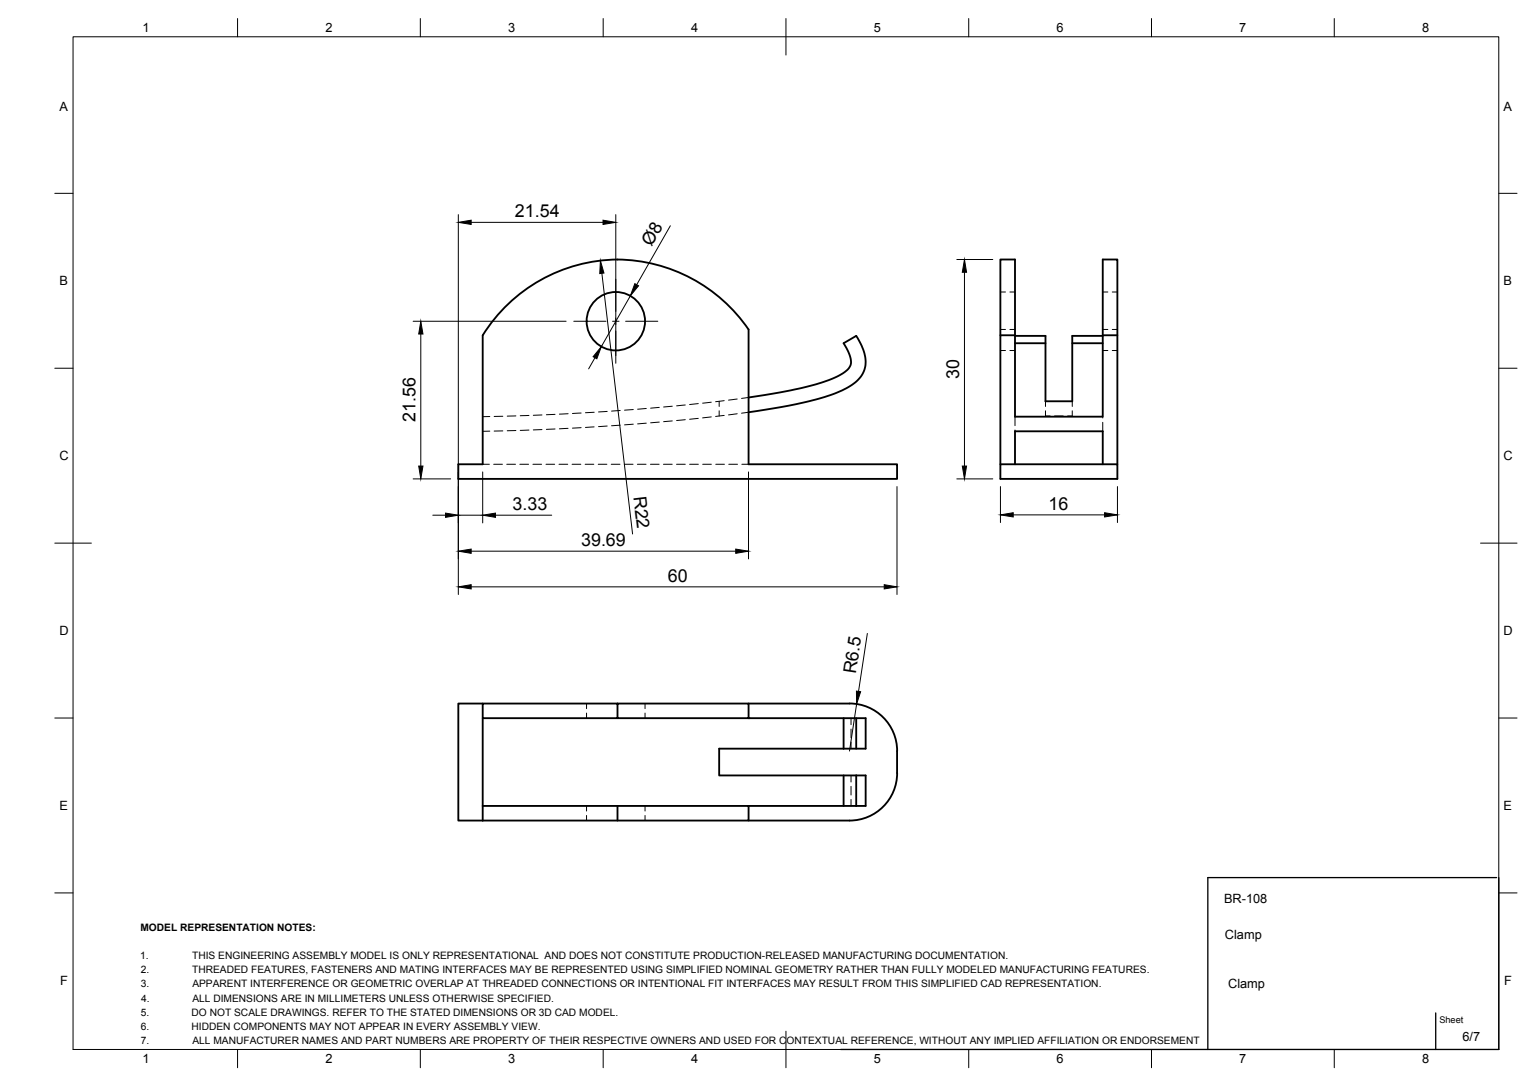
ISO-10303-21;
HEADER;
/* Generated by software containing ST-Developer
 * from STEP Tools, Inc. (www.steptools.com) 
 */

FILE_DESCRIPTION(
/* description */ (''),
/* implementation_level */ '2;1');

FILE_NAME(
/* name */ 'Clamp.step',
/* time_stamp */ '2026-11-14T03:52:36-08:00',
/* author */ (''),
/* organization */ (''),
/* preprocessor_version */ 'ST-DEVELOPER v20.2',
/* originating_system */ 'Autodesk Translation Framework v15.17.0.0',
/* authorisation */ '');

FILE_SCHEMA (('AUTOMOTIVE_DESIGN { 1 0 10303 214 3 1 1 }'));
ENDSEC;

DATA;
#10=MECHANICAL_DESIGN_GEOMETRIC_PRESENTATION_REPRESENTATION('',(#194),#19443);
#45=B_SPLINE_SURFACE_WITH_KNOTS('',5,1,((#10544,#10545),(#10546,#10547),
(#10548,#10549),(#10550,#10551),(#10552,#10553),(#10554,#10555),(#10556,
#10557),(#10558,#10559),(#10560,#10561),(#10562,#10563),(#10564,#10565),
(#10566,#10567),(#10568,#10569),(#10570,#10571),(#10572,#10573),(#10574,
#10575),(#10576,#10577),(#10578,#10579),(#10580,#10581),(#10582,#10583),
(#10584,#10585),(#10586,#10587),(#10588,#10589),(#10590,#10591),(#10592,
#10593)),.UNSPECIFIED.,.F.,.F.,.F.,(6,1,1,1,1,1,1,1,1,1,1,1,1,1,1,1,1,1,
1,1,6),(2,2),(0.,0.05,0.1,0.15,0.2,0.25,0.3,0.35,0.4,0.45,0.5,0.55,0.6,
0.65,0.7,0.75,0.8,0.85,0.9,0.95,0.997783576468117),(0.,2.28),
 .UNSPECIFIED.);
#46=B_SPLINE_SURFACE_WITH_KNOTS('',3,1,((#10795,#10796),(#10797,#10798),
(#10799,#10800),(#10801,#10802),(#10803,#10804),(#10805,#10806),(#10807,
#10808),(#10809,#10810),(#10811,#10812),(#10813,#10814),(#10815,#10816),
(#10817,#10818),(#10819,#10820),(#10821,#10822),(#10823,#10824),(#10825,
#10826),(#10827,#10828),(#10829,#10830),(#10831,#10832),(#10833,#10834),
(#10835,#10836),(#10837,#10838)),.UNSPECIFIED.,.F.,.F.,.F.,(4,3,3,3,3,3,
3,4),(2,2),(-1.,-0.911417181577933,-0.82714074028049,-0.742907558806874,
-0.633245293286216,-0.436057375062027,-0.250000004296482,-0.000486150394329065),
(0.,2.28),.UNSPECIFIED.);
#100=B_SPLINE_CURVE_WITH_KNOTS('',3,(#9842,#9843,#9844,#9845,#9846,#9847,
#9848,#9849,#9850,#9851,#9852,#9853,#9854,#9855,#9856,#9857,#9858,#9859,
#9860,#9861,#9862,#9863,#9864,#9865,#9866,#9867,#9868,#9869,#9870,#9871,
#9872,#9873,#9874,#9875,#9876,#9877,#9878,#9879,#9880,#9881,#9882,#9883,
#9884,#9885,#9886,#9887,#9888,#9889,#9890,#9891,#9892,#9893,#9894,#9895,
#9896,#9897,#9898,#9899,#9900,#9901,#9902,#9903,#9904,#9905,#9906,#9907,
#9908,#9909,#9910,#9911,#9912,#9913,#9914,#9915,#9916,#9917,#9918,#9919,
#9920,#9921,#9922,#9923),.UNSPECIFIED.,.F.,.F.,(4,3,3,3,3,3,3,3,3,3,3,3,
3,3,3,3,3,3,3,3,3,3,3,3,3,3,3,4),(-2.06741991825068,-1.98285131338516,-1.88559013949774,
-1.77615559465644,-1.68790443753717,-1.60974818243148,-1.53676333066918,
-1.46730179083953,-1.4010195987632,-1.3378649598913,-1.27712721666041,-1.21746070099515,
-1.15761317028239,-1.09756920913897,-1.03668973178852,-0.971602936806244,
-0.902947147892858,-0.830652039518071,-0.754808243576467,-0.676131879378777,
-0.596648141755566,-0.518810466257096,-0.437949267560199,-0.352276201339158,
-0.261252153029477,-0.169810646360919,-0.0802964651905899,0.),
 .UNSPECIFIED.);
#101=B_SPLINE_CURVE_WITH_KNOTS('',3,(#9927,#9928,#9929,#9930,#9931,#9932,
#9933,#9934,#9935,#9936,#9937,#9938,#9939,#9940,#9941,#9942,#9943,#9944,
#9945,#9946,#9947,#9948,#9949,#9950,#9951,#9952,#9953,#9954,#9955,#9956,
#9957,#9958,#9959,#9960,#9961,#9962,#9963,#9964,#9965,#9966,#9967,#9968,
#9969,#9970,#9971,#9972,#9973,#9974,#9975,#9976,#9977,#9978,#9979,#9980,
#9981,#9982,#9983,#9984,#9985,#9986,#9987,#9988,#9989,#9990,#9991,#9992,
#9993,#9994,#9995,#9996,#9997,#9998,#9999,#10000,#10001,#10002,#10003,#10004,
#10005,#10006,#10007,#10008,#10009,#10010,#10011,#10012,#10013,#10014,#10015,
#10016,#10017,#10018,#10019,#10020,#10021,#10022,#10023,#10024,#10025,#10026,
#10027,#10028,#10029,#10030,#10031,#10032,#10033,#10034,#10035,#10036,#10037,
#10038,#10039,#10040,#10041,#10042,#10043,#10044,#10045,#10046,#10047,#10048,
#10049,#10050,#10051,#10052,#10053,#10054,#10055,#10056,#10057,#10058,#10059,
#10060,#10061,#10062,#10063,#10064,#10065,#10066,#10067,#10068,#10069,#10070,
#10071,#10072,#10073,#10074,#10075,#10076,#10077,#10078,#10079,#10080,#10081,
#10082,#10083,#10084,#10085,#10086,#10087,#10088,#10089,#10090,#10091,#10092,
#10093,#10094,#10095,#10096,#10097,#10098,#10099,#10100,#10101,#10102,#10103,
#10104,#10105,#10106,#10107,#10108,#10109,#10110,#10111,#10112,#10113,#10114,
#10115,#10116,#10117,#10118,#10119,#10120,#10121,#10122,#10123,#10124,#10125,
#10126,#10127,#10128,#10129,#10130,#10131,#10132,#10133,#10134,#10135,#10136,
#10137,#10138,#10139,#10140,#10141,#10142,#10143,#10144,#10145,#10146,#10147,
#10148,#10149),.UNSPECIFIED.,.F.,.F.,(4,3,3,3,3,3,3,3,3,3,3,3,3,3,3,3,3,
3,3,3,3,3,3,3,3,3,3,3,3,3,3,3,3,3,3,3,3,3,3,3,3,3,3,3,3,3,3,3,3,3,3,3,3,
3,3,3,3,3,3,3,3,3,3,3,3,3,3,3,3,3,3,3,3,3,4),(-5.48556059930356,-5.3742901434944,
-5.26503542580367,-5.1577836872572,-5.04847386928929,-4.94641423339456,
-4.84632584686655,-4.74823870879311,-4.65217176427579,-4.55995510908532,
-4.49079261769247,-4.48335167319748,-4.47546446159234,-4.42482571833493,
-4.37539535138974,-4.32789456523567,-4.28330514351393,-4.22386198589148,
-4.16367959879141,-4.11102001007885,-4.0879814400171,-4.07451117436979,
-4.06881777499082,-4.06396069374141,-4.01960604117804,-3.97171900412971,
-3.91910957291902,-3.86588690476172,-3.81609285440557,-3.7976703630769,
-3.7838534945804,-3.78018597444469,-3.74240288909089,-3.68720132020267,
-3.63214582482016,-3.58397226636046,-3.54161995271181,-3.50476212826565,
-3.48863683007046,-3.48328860908609,-3.47990706616965,-3.42477351581283,
-3.36626643116087,-3.30651189415172,-3.25207197124738,-3.24675735714258,
-3.20212792397615,-3.15620343761748,-3.10888467447819,-3.06005777462237,
-3.00959125336058,-2.9774459670657,-2.96187559401661,-2.95363335797171,
-2.94977181559791,-2.80448949951976,-2.65815449920403,-2.51096234105158,
-2.36291829657365,-2.21466098559846,-2.06653880208347,-1.98094209192433,
-1.80620872497199,-1.61914703673255,-1.40683918645954,-1.18478189892939,
-1.00215186108193,-0.839832576136721,-0.690457992737357,-0.550511129775,
-0.421119097329167,-0.296518986825456,-0.178327808264077,-0.0898716726840916,
-0.0508038206324297),.UNSPECIFIED.);
#102=B_SPLINE_CURVE_WITH_KNOTS('',3,(#10159,#10160,#10161,#10162,#10163,
#10164,#10165,#10166,#10167,#10168,#10169,#10170,#10171,#10172,#10173,#10174,
#10175,#10176,#10177,#10178,#10179,#10180,#10181,#10182,#10183,#10184,#10185,
#10186,#10187,#10188,#10189,#10190,#10191,#10192,#10193,#10194,#10195,#10196,
#10197,#10198,#10199,#10200,#10201,#10202,#10203,#10204,#10205,#10206,#10207,
#10208,#10209,#10210,#10211,#10212,#10213,#10214,#10215,#10216,#10217,#10218,
#10219,#10220,#10221,#10222,#10223,#10224,#10225,#10226,#10227,#10228,#10229,
#10230,#10231,#10232,#10233,#10234,#10235,#10236,#10237,#10238,#10239,#10240,
#10241,#10242,#10243,#10244,#10245,#10246,#10247,#10248,#10249,#10250,#10251,
#10252,#10253,#10254,#10255,#10256,#10257,#10258,#10259,#10260,#10261,#10262,
#10263,#10264,#10265,#10266,#10267,#10268,#10269,#10270,#10271,#10272,#10273,
#10274,#10275,#10276,#10277,#10278,#10279,#10280,#10281,#10282,#10283,#10284,
#10285,#10286,#10287,#10288,#10289,#10290,#10291,#10292,#10293,#10294,#10295,
#10296,#10297,#10298,#10299,#10300,#10301,#10302,#10303,#10304,#10305,#10306),
 .UNSPECIFIED.,.F.,.F.,(4,3,3,3,3,3,3,3,3,3,3,3,3,3,3,3,3,3,3,3,3,3,3,3,
3,3,3,3,3,3,3,3,3,3,3,3,3,3,3,3,3,3,3,3,3,3,3,3,3,4),(-9.10855960492281,
-8.53921958763157,-8.00869400174604,-7.76001013336219,-7.63955388461377,
-7.56405433243604,-7.52369479269779,-7.50080752596703,-7.07650861767828,
-6.72947065932967,-6.625116589863,-6.56600757594707,-6.53309864263095,-6.50820482569483,
-6.14678803531956,-5.8044120104252,-5.71451198234767,-5.68978334933782,
-5.67339715853821,-5.3117835102232,-4.98297267917569,-4.82884260212217,
-4.75418584604937,-4.72996428359645,-4.70456344497697,-4.32299778199833,
-3.91934735473528,-3.47804282231225,-3.37094180328571,-3.35701328282335,
-3.17572752382557,-2.99394470365639,-2.80883622817471,-2.61893869722417,
-2.42004735513258,-2.20439292822488,-1.94398198484001,-1.70733551341788,
-1.50026985092353,-1.31908739624096,-1.16055274839372,-1.01261022609456,
-0.870637451570371,-0.733373124428186,-0.599882166408188,-0.4695171211688,
-0.342516273201481,-0.216889573446191,-0.0922346720977524,-0.0508102134630154),
 .UNSPECIFIED.);
#103=B_SPLINE_CURVE_WITH_KNOTS('',3,(#10309,#10310,#10311,#10312,#10313,
#10314,#10315,#10316,#10317,#10318,#10319,#10320,#10321,#10322,#10323,#10324,
#10325,#10326,#10327,#10328,#10329,#10330,#10331,#10332,#10333,#10334,#10335,
#10336,#10337,#10338,#10339,#10340,#10341,#10342,#10343,#10344,#10345,#10346,
#10347,#10348,#10349,#10350,#10351,#10352,#10353,#10354,#10355,#10356,#10357,
#10358,#10359,#10360,#10361,#10362,#10363,#10364,#10365,#10366,#10367,#10368,
#10369,#10370,#10371,#10372,#10373,#10374,#10375,#10376,#10377,#10378,#10379,
#10380,#10381,#10382,#10383,#10384,#10385,#10386,#10387,#10388,#10389,#10390,
#10391,#10392,#10393,#10394,#10395,#10396,#10397,#10398,#10399,#10400,#10401,
#10402,#10403,#10404,#10405,#10406,#10407,#10408,#10409,#10410,#10411,#10412,
#10413,#10414,#10415,#10416,#10417,#10418,#10419,#10420,#10421,#10422,#10423,
#10424,#10425,#10426,#10427,#10428,#10429,#10430,#10431,#10432,#10433,#10434,
#10435,#10436,#10437,#10438,#10439,#10440,#10441,#10442,#10443,#10444,#10445,
#10446,#10447,#10448,#10449,#10450,#10451,#10452,#10453,#10454,#10455,#10456,
#10457,#10458,#10459,#10460,#10461,#10462,#10463,#10464,#10465,#10466,#10467,
#10468,#10469,#10470,#10471,#10472,#10473,#10474,#10475,#10476,#10477,#10478,
#10479,#10480,#10481,#10482,#10483,#10484,#10485,#10486,#10487,#10488,#10489,
#10490,#10491,#10492,#10493,#10494,#10495,#10496,#10497,#10498,#10499,#10500,
#10501,#10502,#10503,#10504,#10505,#10506,#10507,#10508,#10509,#10510,#10511,
#10512,#10513,#10514,#10515,#10516,#10517,#10518,#10519,#10520,#10521,#10522,
#10523,#10524,#10525,#10526,#10527,#10528,#10529,#10530,#10531,#10532,#10533,
#10534,#10535,#10536,#10537,#10538,#10539,#10540,#10541,#10542,#10543),
 .UNSPECIFIED.,.F.,.F.,(4,3,3,3,3,3,3,3,3,3,3,3,3,3,3,3,3,3,3,3,3,3,3,3,
3,3,3,3,3,3,3,3,3,3,3,3,3,3,3,3,3,3,3,3,3,3,3,3,3,3,3,3,3,3,3,3,3,3,3,3,
3,3,3,3,3,3,3,3,3,3,3,3,3,3,3,3,3,3,4),(-2.02127869660357,-1.98943301980102,
-1.90463341590351,-1.81753768881889,-1.72704367650355,-1.63130693910596,
-1.51951582960439,-1.38310822332673,-1.26646899428466,-1.24459913883927,
-1.23346627262239,-1.22758843562283,-1.22207812234324,-1.15025709426344,
-1.08179540629444,-1.01496797201,-0.950320490610193,-0.916551307158433,
-0.853832223783638,-0.792204136679497,-0.731660192212863,-0.672186959028124,
-0.613766411128121,-0.590013602117237,-0.579621748174975,-0.57475056663954,
-0.571134341312111,-0.569460165760368,-0.547675695632619,-0.526546111795004,
-0.506025620571326,-0.485455200188757,-0.466281411555601,-0.447521496264729,
-0.429320222384578,-0.42374393904105,-0.399392451378572,-0.374499279646305,
-0.361614191206241,-0.358455047560918,-0.356511913591946,-0.35473329500815,
-0.344318954647855,-0.334029402325209,-0.323701337929739,-0.313256768851862,
-0.302559895706747,-0.291964358202782,-0.281691465164288,-0.279957855794893,
-0.278600543326745,-0.271418572125793,-0.262582752193856,-0.253672103340293,
-0.245540273158529,-0.238031151837375,-0.230909539922171,-0.226625838952106,
-0.216671112747294,-0.205500677732474,-0.193363451631138,-0.179480016034121,
-0.176626080324589,-0.166163697812807,-0.160971082256157,-0.159162329434394,
-0.157259342194023,-0.144809310782755,-0.13207070022678,-0.119040767714878,
-0.10571865453773,-0.091955933688298,-0.0779231319105442,-0.0636219003870916,
-0.0490527186804175,-0.034085309706883,-0.0188794529916116,-0.00332468735320998,
0.),.UNSPECIFIED.);
#104=B_SPLINE_CURVE_WITH_KNOTS('',5,(#10597,#10598,#10599,#10600,#10601,
#10602,#10603,#10604,#10605,#10606,#10607,#10608,#10609,#10610,#10611,#10612),
 .UNSPECIFIED.,.F.,.F.,(6,1,1,1,1,1,1,1,1,1,1,6),(0.481836522428161,0.5,
0.55,0.6,0.65,0.7,0.75,0.8,0.85,0.9,0.95,0.997783576468117),
 .UNSPECIFIED.);
#105=B_SPLINE_CURVE_WITH_KNOTS('',5,(#10614,#10615,#10616,#10617,#10618,
#10619,#10620,#10621,#10622,#10623,#10624,#10625,#10626,#10627,#10628),
 .UNSPECIFIED.,.F.,.F.,(6,1,1,1,1,1,1,1,1,1,6),(0.,0.05,0.1,0.15,0.2,0.25,
0.3,0.35,0.4,0.45,0.481836522428277),.UNSPECIFIED.);
#106=B_SPLINE_CURVE_WITH_KNOTS('',3,(#10632,#10633,#10634,#10635,#10636,
#10637,#10638,#10639,#10640,#10641,#10642,#10643,#10644,#10645,#10646,#10647,
#10648,#10649,#10650,#10651,#10652,#10653,#10654,#10655,#10656,#10657,#10658,
#10659,#10660,#10661,#10662,#10663,#10664,#10665,#10666,#10667,#10668,#10669,
#10670,#10671,#10672,#10673,#10674,#10675,#10676,#10677,#10678,#10679,#10680,
#10681,#10682,#10683,#10684,#10685,#10686,#10687,#10688,#10689,#10690,#10691,
#10692,#10693,#10694,#10695),.UNSPECIFIED.,.F.,.F.,(4,3,3,3,3,3,3,3,3,3,
3,3,3,3,3,3,3,3,3,3,3,4),(-0.481836522428277,-0.45532349494856,-0.432546979219204,
-0.411758376367504,-0.392204877029118,-0.373446283655192,-0.35531022111101,
-0.337405801369786,-0.319166348359288,-0.3005346337047,-0.281334526323306,
-0.261758757819788,-0.241752343726884,-0.221237113369723,-0.200124506192356,
-0.178341717407575,-0.155289187104983,-0.131213486522262,-0.105793029252951,
-0.0769868283461338,-0.0445183707397895,0.),.UNSPECIFIED.);
#107=B_SPLINE_CURVE_WITH_KNOTS('',3,(#10697,#10698,#10699,#10700,#10701,
#10702,#10703,#10704,#10705,#10706,#10707,#10708,#10709,#10710,#10711,#10712,
#10713,#10714,#10715,#10716,#10717,#10718,#10719,#10720,#10721,#10722,#10723,
#10724,#10725,#10726,#10727,#10728,#10729,#10730,#10731,#10732,#10733,#10734,
#10735,#10736,#10737,#10738,#10739,#10740,#10741,#10742,#10743,#10744,#10745,
#10746,#10747,#10748,#10749,#10750,#10751,#10752,#10753,#10754,#10755,#10756,
#10757,#10758,#10759,#10760,#10761,#10762,#10763,#10764,#10765,#10766,#10767,
#10768,#10769,#10770,#10771,#10772),.UNSPECIFIED.,.F.,.F.,(4,3,3,3,3,3,
3,3,3,3,3,3,3,3,3,3,3,3,3,3,3,3,3,3,3,4),(-1.78233413254146,-1.68011036101728,
-1.59770235095047,-1.52404961693638,-1.45502228044773,-1.38923460267853,
-1.3265205751834,-1.26669886884287,-1.20909993484359,-1.15227786115506,
-1.09526869988759,-1.03807287674761,-0.979856117355335,-0.917508293433697,
-0.851705632256396,-0.782466326919254,-0.709863093111388,-0.634726037442554,
-0.555385282762235,-0.481050928781323,-0.403338688398482,-0.320930918924746,
-0.234066753872441,-0.147080803661418,-0.0621010514640444,0.),
 .UNSPECIFIED.);
#108=B_SPLINE_CURVE_WITH_KNOTS('',3,(#10782,#10783,#10784,#10785,#10786,
#10787,#10788,#10789,#10790,#10791,#10792,#10793),.UNSPECIFIED.,.F.,.F.,
(4,2,2,2,2,4),(-8.5482923307436,-7.74150904834439,-6.97394683763538,-6.20677862322595,
-5.20801064419706,-3.86462956150548),.UNSPECIFIED.);
#109=B_SPLINE_CURVE_WITH_KNOTS('',3,(#10841,#10842,#10843,#10844,#10845,
#10846,#10847,#10848),.UNSPECIFIED.,.F.,.F.,(4,2,2,4),(0.000486150394328964,
0.250000004296481,0.436057375062024,0.485741739397154),.UNSPECIFIED.);
#110=B_SPLINE_CURVE_WITH_KNOTS('',3,(#10852,#10853,#10854,#10855,#10856,
#10857,#10858,#10859),.UNSPECIFIED.,.F.,.F.,(4,2,2,4),(-0.485741739388686,
-0.436057375062167,-0.250000004296568,-0.000486150394336471),
 .UNSPECIFIED.);
#111=B_SPLINE_CURVE_WITH_KNOTS('',3,(#10860,#10861,#10862,#10863,#10864,
#10865,#10866,#10867,#10868,#10869,#10870,#10871),.UNSPECIFIED.,.F.,.F.,
(4,2,2,2,2,4),(-1.,-0.911417181577934,-0.82714074028049,-0.742907558806875,
-0.633245293286218,-0.485745357261071),.UNSPECIFIED.);
#178=SHAPE_REPRESENTATION_RELATIONSHIP('SRR','None',#19478,#186);
#186=ADVANCED_BREP_SHAPE_REPRESENTATION('',(#202),#19438);
#194=STYLED_ITEM('',(#19525),#202);
#202=MANIFOLD_SOLID_BREP('Body1',#2021);
#210=FACE_BOUND('',#410,.T.);
#211=FACE_BOUND('',#414,.T.);
#212=FACE_BOUND('',#420,.T.);
#213=FACE_BOUND('',#427,.T.);
#227=PLANE('',#2154);
#228=PLANE('',#2158);
#229=PLANE('',#2159);
#230=PLANE('',#2160);
#231=PLANE('',#2161);
#232=PLANE('',#2162);
#233=PLANE('',#2163);
#234=PLANE('',#2164);
#235=PLANE('',#2165);
#236=PLANE('',#2166);
#237=PLANE('',#2167);
#238=PLANE('',#2168);
#239=PLANE('',#2172);
#240=PLANE('',#2173);
#241=PLANE('',#2174);
#242=PLANE('',#2181);
#243=PLANE('',#2182);
#244=PLANE('',#2186);
#245=PLANE('',#2187);
#246=PLANE('',#2194);
#295=FACE_OUTER_BOUND('',#394,.T.);
#296=FACE_OUTER_BOUND('',#395,.T.);
#297=FACE_OUTER_BOUND('',#396,.T.);
#298=FACE_OUTER_BOUND('',#397,.T.);
#299=FACE_OUTER_BOUND('',#398,.T.);
#300=FACE_OUTER_BOUND('',#399,.T.);
#301=FACE_OUTER_BOUND('',#400,.T.);
#302=FACE_OUTER_BOUND('',#401,.T.);
#303=FACE_OUTER_BOUND('',#402,.T.);
#304=FACE_OUTER_BOUND('',#403,.T.);
#305=FACE_OUTER_BOUND('',#404,.T.);
#306=FACE_OUTER_BOUND('',#405,.T.);
#307=FACE_OUTER_BOUND('',#406,.T.);
#308=FACE_OUTER_BOUND('',#407,.T.);
#309=FACE_OUTER_BOUND('',#408,.T.);
#310=FACE_OUTER_BOUND('',#409,.T.);
#311=FACE_OUTER_BOUND('',#411,.T.);
#312=FACE_OUTER_BOUND('',#412,.T.);
#313=FACE_OUTER_BOUND('',#413,.T.);
#314=FACE_OUTER_BOUND('',#415,.T.);
#315=FACE_OUTER_BOUND('',#416,.T.);
#316=FACE_OUTER_BOUND('',#417,.T.);
#317=FACE_OUTER_BOUND('',#418,.T.);
#318=FACE_OUTER_BOUND('',#419,.T.);
#319=FACE_OUTER_BOUND('',#421,.T.);
#320=FACE_OUTER_BOUND('',#422,.T.);
#321=FACE_OUTER_BOUND('',#423,.T.);
#322=FACE_OUTER_BOUND('',#424,.T.);
#323=FACE_OUTER_BOUND('',#425,.T.);
#324=FACE_OUTER_BOUND('',#426,.T.);
#394=EDGE_LOOP('',(#1437,#1438,#1439,#1440));
#395=EDGE_LOOP('',(#1441,#1442,#1443,#1444,#1445,#1446));
#396=EDGE_LOOP('',(#1447,#1448,#1449,#1450));
#397=EDGE_LOOP('',(#1451,#1452,#1453,#1454));
#398=EDGE_LOOP('',(#1455,#1456,#1457,#1458,#1459,#1460,#1461,#1462,#1463,
#1464,#1465,#1466,#1467,#1468));
#399=EDGE_LOOP('',(#1469,#1470,#1471,#1472));
#400=EDGE_LOOP('',(#1473,#1474,#1475,#1476));
#401=EDGE_LOOP('',(#1477,#1478,#1479,#1480));
#402=EDGE_LOOP('',(#1481,#1482,#1483,#1484));
#403=EDGE_LOOP('',(#1485,#1486,#1487,#1488,#1489,#1490,#1491,#1492,#1493,
#1494));
#404=EDGE_LOOP('',(#1495,#1496,#1497,#1498));
#405=EDGE_LOOP('',(#1499,#1500,#1501,#1502));
#406=EDGE_LOOP('',(#1503,#1504,#1505,#1506,#1507,#1508,#1509,#1510,#1511,
#1512));
#407=EDGE_LOOP('',(#1513,#1514,#1515,#1516));
#408=EDGE_LOOP('',(#1517,#1518,#1519,#1520));
#409=EDGE_LOOP('',(#1521,#1522,#1523,#1524,#1525));
#410=EDGE_LOOP('',(#1526));
#411=EDGE_LOOP('',(#1527,#1528,#1529,#1530));
#412=EDGE_LOOP('',(#1531,#1532,#1533,#1534,#1535,#1536));
#413=EDGE_LOOP('',(#1537,#1538,#1539,#1540,#1541,#1542,#1543,#1544,#1545));
#414=EDGE_LOOP('',(#1546));
#415=EDGE_LOOP('',(#1547,#1548,#1549,#1550));
#416=EDGE_LOOP('',(#1551,#1552,#1553,#1554));
#417=EDGE_LOOP('',(#1555,#1556,#1557,#1558));
#418=EDGE_LOOP('',(#1559,#1560,#1561,#1562));
#419=EDGE_LOOP('',(#1563,#1564,#1565,#1566,#1567));
#420=EDGE_LOOP('',(#1568));
#421=EDGE_LOOP('',(#1569,#1570,#1571,#1572,#1573,#1574,#1575,#1576,#1577,
#1578,#1579,#1580));
#422=EDGE_LOOP('',(#1581,#1582,#1583,#1584,#1585,#1586));
#423=EDGE_LOOP('',(#1587,#1588,#1589,#1590));
#424=EDGE_LOOP('',(#1591,#1592,#1593,#1594));
#425=EDGE_LOOP('',(#1595,#1596,#1597,#1598));
#426=EDGE_LOOP('',(#1599,#1600,#1601,#1602,#1603,#1604,#1605,#1606,#1607));
#427=EDGE_LOOP('',(#1608));
#489=LINE('',#9792,#616);
#490=LINE('',#9795,#617);
#491=LINE('',#9798,#618);
#492=LINE('',#9802,#619);
#493=LINE('',#9804,#620);
#494=LINE('',#9805,#621);
#495=LINE('',#9808,#622);
#496=LINE('',#9811,#623);
#497=LINE('',#9813,#624);
#498=LINE('',#9817,#625);
#499=LINE('',#9818,#626);
#500=LINE('',#9820,#627);
#501=LINE('',#9822,#628);
#502=LINE('',#9824,#629);
#503=LINE('',#9826,#630);
#504=LINE('',#9828,#631);
#505=LINE('',#9830,#632);
#506=LINE('',#9832,#633);
#507=LINE('',#9834,#634);
#508=LINE('',#9835,#635);
#509=LINE('',#9837,#636);
#510=LINE('',#9838,#637);
#511=LINE('',#9925,#638);
#512=LINE('',#10150,#639);
#513=LINE('',#10153,#640);
#514=LINE('',#10155,#641);
#515=LINE('',#10156,#642);
#516=LINE('',#10308,#643);
#517=LINE('',#10595,#644);
#518=LINE('',#10630,#645);
#519=LINE('',#10773,#646);
#520=LINE('',#10776,#647);
#521=LINE('',#10777,#648);
#522=LINE('',#10780,#649);
#523=LINE('',#10794,#650);
#524=LINE('',#10839,#651);
#525=LINE('',#10850,#652);
#526=LINE('',#10874,#653);
#527=LINE('',#10877,#654);
#528=LINE('',#10882,#655);
#529=LINE('',#10886,#656);
#530=LINE('',#10887,#657);
#531=LINE('',#10890,#658);
#532=LINE('',#10891,#659);
#533=LINE('',#10894,#660);
#534=LINE('',#10901,#661);
#535=LINE('',#10903,#662);
#536=LINE('',#10905,#663);
#537=LINE('',#10907,#664);
#538=LINE('',#10908,#665);
#539=LINE('',#10911,#666);
#540=LINE('',#10916,#667);
#541=LINE('',#10921,#668);
#542=LINE('',#10922,#669);
#543=LINE('',#10925,#670);
#544=LINE('',#10926,#671);
#545=LINE('',#10930,#672);
#546=LINE('',#10934,#673);
#616=VECTOR('',#2353,10.);
#617=VECTOR('',#2356,10.);
#618=VECTOR('',#2359,10.);
#619=VECTOR('',#2362,10.);
#620=VECTOR('',#2363,10.);
#621=VECTOR('',#2364,10.);
#622=VECTOR('',#2367,10.);
#623=VECTOR('',#2370,10.);
#624=VECTOR('',#2373,10.);
#625=VECTOR('',#2376,10.);
#626=VECTOR('',#2377,10.);
#627=VECTOR('',#2378,10.);
#628=VECTOR('',#2379,10.);
#629=VECTOR('',#2380,10.);
#630=VECTOR('',#2381,10.);
#631=VECTOR('',#2382,10.);
#632=VECTOR('',#2383,10.);
#633=VECTOR('',#2384,10.);
#634=VECTOR('',#2385,10.);
#635=VECTOR('',#2386,10.);
#636=VECTOR('',#2389,10.);
#637=VECTOR('',#2390,10.);
#638=VECTOR('',#2393,10.);
#639=VECTOR('',#2394,10.);
#640=VECTOR('',#2397,10.);
#641=VECTOR('',#2398,10.);
#642=VECTOR('',#2399,10.);
#643=VECTOR('',#2402,10.);
#644=VECTOR('',#2403,10.);
#645=VECTOR('',#2404,10.);
#646=VECTOR('',#2405,10.);
#647=VECTOR('',#2408,10.);
#648=VECTOR('',#2409,10.);
#649=VECTOR('',#2412,10.);
#650=VECTOR('',#2413,10.);
#651=VECTOR('',#2414,10.);
#652=VECTOR('',#2415,10.);
#653=VECTOR('',#2420,10.);
#654=VECTOR('',#2423,10.);
#655=VECTOR('',#2428,10.);
#656=VECTOR('',#2433,10.);
#657=VECTOR('',#2434,10.);
#658=VECTOR('',#2437,10.);
#659=VECTOR('',#2438,10.);
#660=VECTOR('',#2441,10.);
#661=VECTOR('',#2450,3.99999999999997);
#662=VECTOR('',#2453,10.);
#663=VECTOR('',#2456,10.);
#664=VECTOR('',#2459,10.);
#665=VECTOR('',#2460,10.);
#666=VECTOR('',#2463,10.);
#667=VECTOR('',#2468,10.);
#668=VECTOR('',#2473,10.);
#669=VECTOR('',#2474,10.);
#670=VECTOR('',#2477,10.);
#671=VECTOR('',#2478,10.);
#672=VECTOR('',#2483,3.99999999999997);
#673=VECTOR('',#2488,10.);
#743=CIRCLE('',#2152,6.5);
#744=CIRCLE('',#2153,6.5);
#745=CIRCLE('',#2155,6.5);
#746=CIRCLE('',#2157,6.5);
#747=CIRCLE('',#2169,22.);
#748=CIRCLE('',#2170,22.);
#749=CIRCLE('',#2171,3.99999999999997);
#750=CIRCLE('',#2175,22.);
#751=CIRCLE('',#2176,22.);
#752=CIRCLE('',#2177,3.99999999999997);
#753=CIRCLE('',#2183,22.);
#754=CIRCLE('',#2184,22.);
#755=CIRCLE('',#2185,3.99999999999997);
#756=CIRCLE('',#2189,3.99999999999997);
#757=CIRCLE('',#2191,22.);
#758=CIRCLE('',#2193,22.);
#834=VERTEX_POINT('',#9788);
#835=VERTEX_POINT('',#9789);
#836=VERTEX_POINT('',#9791);
#837=VERTEX_POINT('',#9793);
#838=VERTEX_POINT('',#9797);
#839=VERTEX_POINT('',#9799);
#840=VERTEX_POINT('',#9801);
#841=VERTEX_POINT('',#9803);
#842=VERTEX_POINT('',#9807);
#843=VERTEX_POINT('',#9809);
#844=VERTEX_POINT('',#9815);
#845=VERTEX_POINT('',#9816);
#846=VERTEX_POINT('',#9819);
#847=VERTEX_POINT('',#9821);
#848=VERTEX_POINT('',#9823);
#849=VERTEX_POINT('',#9825);
#850=VERTEX_POINT('',#9827);
#851=VERTEX_POINT('',#9829);
#852=VERTEX_POINT('',#9831);
#853=VERTEX_POINT('',#9833);
#854=VERTEX_POINT('',#9840);
#855=VERTEX_POINT('',#9841);
#856=VERTEX_POINT('',#9924);
#857=VERTEX_POINT('',#9926);
#858=VERTEX_POINT('',#10152);
#859=VERTEX_POINT('',#10154);
#860=VERTEX_POINT('',#10158);
#861=VERTEX_POINT('',#10307);
#862=VERTEX_POINT('',#10594);
#863=VERTEX_POINT('',#10596);
#864=VERTEX_POINT('',#10613);
#865=VERTEX_POINT('',#10629);
#866=VERTEX_POINT('',#10631);
#867=VERTEX_POINT('',#10696);
#868=VERTEX_POINT('',#10775);
#869=VERTEX_POINT('',#10779);
#870=VERTEX_POINT('',#10781);
#871=VERTEX_POINT('',#10840);
#872=VERTEX_POINT('',#10849);
#873=VERTEX_POINT('',#10851);
#874=VERTEX_POINT('',#10876);
#875=VERTEX_POINT('',#10878);
#876=VERTEX_POINT('',#10880);
#877=VERTEX_POINT('',#10883);
#878=VERTEX_POINT('',#10889);
#879=VERTEX_POINT('',#10893);
#880=VERTEX_POINT('',#10895);
#881=VERTEX_POINT('',#10898);
#882=VERTEX_POINT('',#10910);
#883=VERTEX_POINT('',#10912);
#884=VERTEX_POINT('',#10914);
#885=VERTEX_POINT('',#10917);
#886=VERTEX_POINT('',#10920);
#887=VERTEX_POINT('',#10924);
#888=VERTEX_POINT('',#10928);
#889=VERTEX_POINT('',#10932);
#1067=EDGE_CURVE('',#834,#835,#743,.T.);
#1068=EDGE_CURVE('',#835,#836,#489,.T.);
#1069=EDGE_CURVE('',#836,#837,#744,.T.);
#1070=EDGE_CURVE('',#837,#834,#490,.T.);
#1071=EDGE_CURVE('',#834,#838,#491,.T.);
#1072=EDGE_CURVE('',#839,#838,#745,.T.);
#1073=EDGE_CURVE('',#839,#840,#492,.T.);
#1074=EDGE_CURVE('',#841,#840,#493,.T.);
#1075=EDGE_CURVE('',#835,#841,#494,.T.);
#1076=EDGE_CURVE('',#838,#842,#495,.T.);
#1077=EDGE_CURVE('',#842,#843,#746,.T.);
#1078=EDGE_CURVE('',#843,#839,#496,.T.);
#1079=EDGE_CURVE('',#837,#842,#497,.T.);
#1080=EDGE_CURVE('',#844,#845,#498,.T.);
#1081=EDGE_CURVE('',#845,#843,#499,.T.);
#1082=EDGE_CURVE('',#846,#836,#500,.T.);
#1083=EDGE_CURVE('',#846,#847,#501,.T.);
#1084=EDGE_CURVE('',#848,#847,#502,.T.);
#1085=EDGE_CURVE('',#848,#849,#503,.T.);
#1086=EDGE_CURVE('',#850,#849,#504,.T.);
#1087=EDGE_CURVE('',#851,#850,#505,.T.);
#1088=EDGE_CURVE('',#851,#852,#506,.T.);
#1089=EDGE_CURVE('',#852,#853,#507,.T.);
#1090=EDGE_CURVE('',#844,#853,#508,.T.);
#1091=EDGE_CURVE('',#841,#850,#509,.T.);
#1092=EDGE_CURVE('',#840,#851,#510,.T.);
#1093=EDGE_CURVE('',#854,#855,#100,.T.);
#1094=EDGE_CURVE('',#854,#856,#511,.T.);
#1095=EDGE_CURVE('',#857,#856,#101,.T.);
#1096=EDGE_CURVE('',#855,#857,#512,.T.);
#1097=EDGE_CURVE('',#858,#854,#513,.T.);
#1098=EDGE_CURVE('',#858,#859,#514,.T.);
#1099=EDGE_CURVE('',#856,#859,#515,.T.);
#1100=EDGE_CURVE('',#860,#858,#102,.T.);
#1101=EDGE_CURVE('',#861,#860,#516,.T.);
#1102=EDGE_CURVE('',#859,#861,#103,.T.);
#1103=EDGE_CURVE('',#855,#862,#517,.T.);
#1104=EDGE_CURVE('',#863,#862,#104,.T.);
#1105=EDGE_CURVE('',#864,#863,#105,.T.);
#1106=EDGE_CURVE('',#865,#864,#518,.T.);
#1107=EDGE_CURVE('',#866,#865,#106,.T.);
#1108=EDGE_CURVE('',#866,#867,#107,.T.);
#1109=EDGE_CURVE('',#867,#860,#519,.T.);
#1110=EDGE_CURVE('',#857,#868,#520,.T.);
#1111=EDGE_CURVE('',#862,#868,#521,.T.);
#1112=EDGE_CURVE('',#866,#869,#522,.T.);
#1113=EDGE_CURVE('',#870,#869,#108,.T.);
#1114=EDGE_CURVE('',#867,#870,#523,.T.);
#1115=EDGE_CURVE('',#870,#861,#524,.T.);
#1116=EDGE_CURVE('',#871,#869,#109,.T.);
#1117=EDGE_CURVE('',#871,#872,#525,.T.);
#1118=EDGE_CURVE('',#873,#872,#110,.T.);
#1119=EDGE_CURVE('',#868,#873,#111,.T.);
#1120=EDGE_CURVE('',#873,#863,#526,.T.);
#1121=EDGE_CURVE('',#872,#874,#527,.T.);
#1122=EDGE_CURVE('',#875,#874,#747,.T.);
#1123=EDGE_CURVE('',#876,#875,#748,.T.);
#1124=EDGE_CURVE('',#876,#873,#528,.T.);
#1125=EDGE_CURVE('',#877,#877,#749,.T.);
#1126=EDGE_CURVE('',#863,#844,#529,.T.);
#1127=EDGE_CURVE('',#853,#864,#530,.T.);
#1128=EDGE_CURVE('',#878,#876,#531,.T.);
#1129=EDGE_CURVE('',#845,#878,#532,.T.);
#1130=EDGE_CURVE('',#879,#852,#533,.T.);
#1131=EDGE_CURVE('',#878,#880,#750,.T.);
#1132=EDGE_CURVE('',#880,#879,#751,.T.);
#1133=EDGE_CURVE('',#881,#881,#752,.T.);
#1134=EDGE_CURVE('',#877,#881,#534,.T.);
#1135=EDGE_CURVE('',#875,#880,#535,.T.);
#1136=EDGE_CURVE('',#874,#879,#536,.T.);
#1137=EDGE_CURVE('',#865,#848,#537,.T.);
#1138=EDGE_CURVE('',#847,#866,#538,.T.);
#1139=EDGE_CURVE('',#869,#882,#539,.T.);
#1140=EDGE_CURVE('',#882,#883,#753,.T.);
#1141=EDGE_CURVE('',#883,#884,#754,.T.);
#1142=EDGE_CURVE('',#884,#871,#540,.T.);
#1143=EDGE_CURVE('',#885,#885,#755,.T.);
#1144=EDGE_CURVE('',#886,#884,#541,.T.);
#1145=EDGE_CURVE('',#849,#886,#542,.T.);
#1146=EDGE_CURVE('',#887,#846,#543,.T.);
#1147=EDGE_CURVE('',#882,#887,#544,.T.);
#1148=EDGE_CURVE('',#888,#888,#756,.T.);
#1149=EDGE_CURVE('',#888,#885,#545,.T.);
#1150=EDGE_CURVE('',#887,#889,#757,.T.);
#1151=EDGE_CURVE('',#889,#883,#546,.T.);
#1152=EDGE_CURVE('',#889,#886,#758,.T.);
#1437=ORIENTED_EDGE('',*,*,#1067,.T.);
#1438=ORIENTED_EDGE('',*,*,#1068,.T.);
#1439=ORIENTED_EDGE('',*,*,#1069,.T.);
#1440=ORIENTED_EDGE('',*,*,#1070,.T.);
#1441=ORIENTED_EDGE('',*,*,#1067,.F.);
#1442=ORIENTED_EDGE('',*,*,#1071,.T.);
#1443=ORIENTED_EDGE('',*,*,#1072,.F.);
#1444=ORIENTED_EDGE('',*,*,#1073,.T.);
#1445=ORIENTED_EDGE('',*,*,#1074,.F.);
#1446=ORIENTED_EDGE('',*,*,#1075,.F.);
#1447=ORIENTED_EDGE('',*,*,#1072,.T.);
#1448=ORIENTED_EDGE('',*,*,#1076,.T.);
#1449=ORIENTED_EDGE('',*,*,#1077,.T.);
#1450=ORIENTED_EDGE('',*,*,#1078,.T.);
#1451=ORIENTED_EDGE('',*,*,#1070,.F.);
#1452=ORIENTED_EDGE('',*,*,#1079,.T.);
#1453=ORIENTED_EDGE('',*,*,#1076,.F.);
#1454=ORIENTED_EDGE('',*,*,#1071,.F.);
#1455=ORIENTED_EDGE('',*,*,#1080,.T.);
#1456=ORIENTED_EDGE('',*,*,#1081,.T.);
#1457=ORIENTED_EDGE('',*,*,#1077,.F.);
#1458=ORIENTED_EDGE('',*,*,#1079,.F.);
#1459=ORIENTED_EDGE('',*,*,#1069,.F.);
#1460=ORIENTED_EDGE('',*,*,#1082,.F.);
#1461=ORIENTED_EDGE('',*,*,#1083,.T.);
#1462=ORIENTED_EDGE('',*,*,#1084,.F.);
#1463=ORIENTED_EDGE('',*,*,#1085,.T.);
#1464=ORIENTED_EDGE('',*,*,#1086,.F.);
#1465=ORIENTED_EDGE('',*,*,#1087,.F.);
#1466=ORIENTED_EDGE('',*,*,#1088,.T.);
#1467=ORIENTED_EDGE('',*,*,#1089,.T.);
#1468=ORIENTED_EDGE('',*,*,#1090,.F.);
#1469=ORIENTED_EDGE('',*,*,#1087,.T.);
#1470=ORIENTED_EDGE('',*,*,#1091,.F.);
#1471=ORIENTED_EDGE('',*,*,#1074,.T.);
#1472=ORIENTED_EDGE('',*,*,#1092,.T.);
#1473=ORIENTED_EDGE('',*,*,#1093,.F.);
#1474=ORIENTED_EDGE('',*,*,#1094,.T.);
#1475=ORIENTED_EDGE('',*,*,#1095,.F.);
#1476=ORIENTED_EDGE('',*,*,#1096,.F.);
#1477=ORIENTED_EDGE('',*,*,#1097,.F.);
#1478=ORIENTED_EDGE('',*,*,#1098,.T.);
#1479=ORIENTED_EDGE('',*,*,#1099,.F.);
#1480=ORIENTED_EDGE('',*,*,#1094,.F.);
#1481=ORIENTED_EDGE('',*,*,#1100,.F.);
#1482=ORIENTED_EDGE('',*,*,#1101,.F.);
#1483=ORIENTED_EDGE('',*,*,#1102,.F.);
#1484=ORIENTED_EDGE('',*,*,#1098,.F.);
#1485=ORIENTED_EDGE('',*,*,#1100,.T.);
#1486=ORIENTED_EDGE('',*,*,#1097,.T.);
#1487=ORIENTED_EDGE('',*,*,#1093,.T.);
#1488=ORIENTED_EDGE('',*,*,#1103,.T.);
#1489=ORIENTED_EDGE('',*,*,#1104,.F.);
#1490=ORIENTED_EDGE('',*,*,#1105,.F.);
#1491=ORIENTED_EDGE('',*,*,#1106,.F.);
#1492=ORIENTED_EDGE('',*,*,#1107,.F.);
#1493=ORIENTED_EDGE('',*,*,#1108,.T.);
#1494=ORIENTED_EDGE('',*,*,#1109,.T.);
#1495=ORIENTED_EDGE('',*,*,#1096,.T.);
#1496=ORIENTED_EDGE('',*,*,#1110,.T.);
#1497=ORIENTED_EDGE('',*,*,#1111,.F.);
#1498=ORIENTED_EDGE('',*,*,#1103,.F.);
#1499=ORIENTED_EDGE('',*,*,#1112,.T.);
#1500=ORIENTED_EDGE('',*,*,#1113,.F.);
#1501=ORIENTED_EDGE('',*,*,#1114,.F.);
#1502=ORIENTED_EDGE('',*,*,#1108,.F.);
#1503=ORIENTED_EDGE('',*,*,#1102,.T.);
#1504=ORIENTED_EDGE('',*,*,#1115,.F.);
#1505=ORIENTED_EDGE('',*,*,#1113,.T.);
#1506=ORIENTED_EDGE('',*,*,#1116,.F.);
#1507=ORIENTED_EDGE('',*,*,#1117,.T.);
#1508=ORIENTED_EDGE('',*,*,#1118,.F.);
#1509=ORIENTED_EDGE('',*,*,#1119,.F.);
#1510=ORIENTED_EDGE('',*,*,#1110,.F.);
#1511=ORIENTED_EDGE('',*,*,#1095,.T.);
#1512=ORIENTED_EDGE('',*,*,#1099,.T.);
#1513=ORIENTED_EDGE('',*,*,#1101,.T.);
#1514=ORIENTED_EDGE('',*,*,#1109,.F.);
#1515=ORIENTED_EDGE('',*,*,#1114,.T.);
#1516=ORIENTED_EDGE('',*,*,#1115,.T.);
#1517=ORIENTED_EDGE('',*,*,#1120,.T.);
#1518=ORIENTED_EDGE('',*,*,#1104,.T.);
#1519=ORIENTED_EDGE('',*,*,#1111,.T.);
#1520=ORIENTED_EDGE('',*,*,#1119,.T.);
#1521=ORIENTED_EDGE('',*,*,#1118,.T.);
#1522=ORIENTED_EDGE('',*,*,#1121,.T.);
#1523=ORIENTED_EDGE('',*,*,#1122,.F.);
#1524=ORIENTED_EDGE('',*,*,#1123,.F.);
#1525=ORIENTED_EDGE('',*,*,#1124,.T.);
#1526=ORIENTED_EDGE('',*,*,#1125,.F.);
#1527=ORIENTED_EDGE('',*,*,#1105,.T.);
#1528=ORIENTED_EDGE('',*,*,#1126,.T.);
#1529=ORIENTED_EDGE('',*,*,#1090,.T.);
#1530=ORIENTED_EDGE('',*,*,#1127,.T.);
#1531=ORIENTED_EDGE('',*,*,#1124,.F.);
#1532=ORIENTED_EDGE('',*,*,#1128,.F.);
#1533=ORIENTED_EDGE('',*,*,#1129,.F.);
#1534=ORIENTED_EDGE('',*,*,#1080,.F.);
#1535=ORIENTED_EDGE('',*,*,#1126,.F.);
#1536=ORIENTED_EDGE('',*,*,#1120,.F.);
#1537=ORIENTED_EDGE('',*,*,#1130,.T.);
#1538=ORIENTED_EDGE('',*,*,#1088,.F.);
#1539=ORIENTED_EDGE('',*,*,#1092,.F.);
#1540=ORIENTED_EDGE('',*,*,#1073,.F.);
#1541=ORIENTED_EDGE('',*,*,#1078,.F.);
#1542=ORIENTED_EDGE('',*,*,#1081,.F.);
#1543=ORIENTED_EDGE('',*,*,#1129,.T.);
#1544=ORIENTED_EDGE('',*,*,#1131,.T.);
#1545=ORIENTED_EDGE('',*,*,#1132,.T.);
#1546=ORIENTED_EDGE('',*,*,#1133,.T.);
#1547=ORIENTED_EDGE('',*,*,#1125,.T.);
#1548=ORIENTED_EDGE('',*,*,#1134,.T.);
#1549=ORIENTED_EDGE('',*,*,#1133,.F.);
#1550=ORIENTED_EDGE('',*,*,#1134,.F.);
#1551=ORIENTED_EDGE('',*,*,#1128,.T.);
#1552=ORIENTED_EDGE('',*,*,#1123,.T.);
#1553=ORIENTED_EDGE('',*,*,#1135,.T.);
#1554=ORIENTED_EDGE('',*,*,#1131,.F.);
#1555=ORIENTED_EDGE('',*,*,#1136,.T.);
#1556=ORIENTED_EDGE('',*,*,#1132,.F.);
#1557=ORIENTED_EDGE('',*,*,#1135,.F.);
#1558=ORIENTED_EDGE('',*,*,#1122,.T.);
#1559=ORIENTED_EDGE('',*,*,#1107,.T.);
#1560=ORIENTED_EDGE('',*,*,#1137,.T.);
#1561=ORIENTED_EDGE('',*,*,#1084,.T.);
#1562=ORIENTED_EDGE('',*,*,#1138,.T.);
#1563=ORIENTED_EDGE('',*,*,#1116,.T.);
#1564=ORIENTED_EDGE('',*,*,#1139,.T.);
#1565=ORIENTED_EDGE('',*,*,#1140,.T.);
#1566=ORIENTED_EDGE('',*,*,#1141,.T.);
#1567=ORIENTED_EDGE('',*,*,#1142,.T.);
#1568=ORIENTED_EDGE('',*,*,#1143,.T.);
#1569=ORIENTED_EDGE('',*,*,#1142,.F.);
#1570=ORIENTED_EDGE('',*,*,#1144,.F.);
#1571=ORIENTED_EDGE('',*,*,#1145,.F.);
#1572=ORIENTED_EDGE('',*,*,#1085,.F.);
#1573=ORIENTED_EDGE('',*,*,#1137,.F.);
#1574=ORIENTED_EDGE('',*,*,#1106,.T.);
#1575=ORIENTED_EDGE('',*,*,#1127,.F.);
#1576=ORIENTED_EDGE('',*,*,#1089,.F.);
#1577=ORIENTED_EDGE('',*,*,#1130,.F.);
#1578=ORIENTED_EDGE('',*,*,#1136,.F.);
#1579=ORIENTED_EDGE('',*,*,#1121,.F.);
#1580=ORIENTED_EDGE('',*,*,#1117,.F.);
#1581=ORIENTED_EDGE('',*,*,#1138,.F.);
#1582=ORIENTED_EDGE('',*,*,#1083,.F.);
#1583=ORIENTED_EDGE('',*,*,#1146,.F.);
#1584=ORIENTED_EDGE('',*,*,#1147,.F.);
#1585=ORIENTED_EDGE('',*,*,#1139,.F.);
#1586=ORIENTED_EDGE('',*,*,#1112,.F.);
#1587=ORIENTED_EDGE('',*,*,#1148,.T.);
#1588=ORIENTED_EDGE('',*,*,#1149,.T.);
#1589=ORIENTED_EDGE('',*,*,#1143,.F.);
#1590=ORIENTED_EDGE('',*,*,#1149,.F.);
#1591=ORIENTED_EDGE('',*,*,#1147,.T.);
#1592=ORIENTED_EDGE('',*,*,#1150,.T.);
#1593=ORIENTED_EDGE('',*,*,#1151,.T.);
#1594=ORIENTED_EDGE('',*,*,#1140,.F.);
#1595=ORIENTED_EDGE('',*,*,#1144,.T.);
#1596=ORIENTED_EDGE('',*,*,#1141,.F.);
#1597=ORIENTED_EDGE('',*,*,#1151,.F.);
#1598=ORIENTED_EDGE('',*,*,#1152,.T.);
#1599=ORIENTED_EDGE('',*,*,#1145,.T.);
#1600=ORIENTED_EDGE('',*,*,#1152,.F.);
#1601=ORIENTED_EDGE('',*,*,#1150,.F.);
#1602=ORIENTED_EDGE('',*,*,#1146,.T.);
#1603=ORIENTED_EDGE('',*,*,#1082,.T.);
#1604=ORIENTED_EDGE('',*,*,#1068,.F.);
#1605=ORIENTED_EDGE('',*,*,#1075,.T.);
#1606=ORIENTED_EDGE('',*,*,#1091,.T.);
#1607=ORIENTED_EDGE('',*,*,#1086,.T.);
#1608=ORIENTED_EDGE('',*,*,#1148,.F.);
#1898=CYLINDRICAL_SURFACE('',#2151,6.5);
#1899=CYLINDRICAL_SURFACE('',#2156,6.5);
#1900=CYLINDRICAL_SURFACE('',#2178,3.99999999999997);
#1901=CYLINDRICAL_SURFACE('',#2179,22.);
#1902=CYLINDRICAL_SURFACE('',#2180,22.);
#1903=CYLINDRICAL_SURFACE('',#2188,3.99999999999997);
#1904=CYLINDRICAL_SURFACE('',#2190,22.);
#1905=CYLINDRICAL_SURFACE('',#2192,22.);
#1944=ADVANCED_FACE('',(#295),#1898,.T.);
#1945=ADVANCED_FACE('',(#296),#227,.T.);
#1946=ADVANCED_FACE('',(#297),#1899,.T.);
#1947=ADVANCED_FACE('',(#298),#228,.T.);
#1948=ADVANCED_FACE('',(#299),#229,.T.);
#1949=ADVANCED_FACE('',(#300),#230,.T.);
#1950=ADVANCED_FACE('',(#301),#231,.F.);
#1951=ADVANCED_FACE('',(#302),#232,.F.);
#1952=ADVANCED_FACE('',(#303),#233,.F.);
#1953=ADVANCED_FACE('',(#304),#45,.T.);
#1954=ADVANCED_FACE('',(#305),#234,.T.);
#1955=ADVANCED_FACE('',(#306),#235,.F.);
#1956=ADVANCED_FACE('',(#307),#46,.T.);
#1957=ADVANCED_FACE('',(#308),#236,.T.);
#1958=ADVANCED_FACE('',(#309),#237,.T.);
#1959=ADVANCED_FACE('',(#310,#210),#238,.F.);
#1960=ADVANCED_FACE('',(#311),#239,.F.);
#1961=ADVANCED_FACE('',(#312),#240,.F.);
#1962=ADVANCED_FACE('',(#313,#211),#241,.T.);
#1963=ADVANCED_FACE('',(#314),#1900,.F.);
#1964=ADVANCED_FACE('',(#315),#1901,.T.);
#1965=ADVANCED_FACE('',(#316),#1902,.T.);
#1966=ADVANCED_FACE('',(#317),#242,.T.);
#1967=ADVANCED_FACE('',(#318,#212),#243,.T.);
#1968=ADVANCED_FACE('',(#319),#244,.F.);
#1969=ADVANCED_FACE('',(#320),#245,.F.);
#1970=ADVANCED_FACE('',(#321),#1903,.F.);
#1971=ADVANCED_FACE('',(#322),#1904,.T.);
#1972=ADVANCED_FACE('',(#323),#1905,.T.);
#1973=ADVANCED_FACE('',(#324,#213),#246,.F.);
#2021=CLOSED_SHELL('',(#1944,#1945,#1946,#1947,#1948,#1949,#1950,#1951,
#1952,#1953,#1954,#1955,#1956,#1957,#1958,#1959,#1960,#1961,#1962,#1963,
#1964,#1965,#1966,#1967,#1968,#1969,#1970,#1971,#1972,#1973));
#2150=AXIS2_PLACEMENT_3D('',#9786,#2347,#2348);
#2151=AXIS2_PLACEMENT_3D('',#9787,#2349,#2350);
#2152=AXIS2_PLACEMENT_3D('',#9790,#2351,#2352);
#2153=AXIS2_PLACEMENT_3D('',#9794,#2354,#2355);
#2154=AXIS2_PLACEMENT_3D('',#9796,#2357,#2358);
#2155=AXIS2_PLACEMENT_3D('',#9800,#2360,#2361);
#2156=AXIS2_PLACEMENT_3D('',#9806,#2365,#2366);
#2157=AXIS2_PLACEMENT_3D('',#9810,#2368,#2369);
#2158=AXIS2_PLACEMENT_3D('',#9812,#2371,#2372);
#2159=AXIS2_PLACEMENT_3D('',#9814,#2374,#2375);
#2160=AXIS2_PLACEMENT_3D('',#9836,#2387,#2388);
#2161=AXIS2_PLACEMENT_3D('',#9839,#2391,#2392);
#2162=AXIS2_PLACEMENT_3D('',#10151,#2395,#2396);
#2163=AXIS2_PLACEMENT_3D('',#10157,#2400,#2401);
#2164=AXIS2_PLACEMENT_3D('',#10774,#2406,#2407);
#2165=AXIS2_PLACEMENT_3D('',#10778,#2410,#2411);
#2166=AXIS2_PLACEMENT_3D('',#10872,#2416,#2417);
#2167=AXIS2_PLACEMENT_3D('',#10873,#2418,#2419);
#2168=AXIS2_PLACEMENT_3D('',#10875,#2421,#2422);
#2169=AXIS2_PLACEMENT_3D('',#10879,#2424,#2425);
#2170=AXIS2_PLACEMENT_3D('',#10881,#2426,#2427);
#2171=AXIS2_PLACEMENT_3D('',#10884,#2429,#2430);
#2172=AXIS2_PLACEMENT_3D('',#10885,#2431,#2432);
#2173=AXIS2_PLACEMENT_3D('',#10888,#2435,#2436);
#2174=AXIS2_PLACEMENT_3D('',#10892,#2439,#2440);
#2175=AXIS2_PLACEMENT_3D('',#10896,#2442,#2443);
#2176=AXIS2_PLACEMENT_3D('',#10897,#2444,#2445);
#2177=AXIS2_PLACEMENT_3D('',#10899,#2446,#2447);
#2178=AXIS2_PLACEMENT_3D('',#10900,#2448,#2449);
#2179=AXIS2_PLACEMENT_3D('',#10902,#2451,#2452);
#2180=AXIS2_PLACEMENT_3D('',#10904,#2454,#2455);
#2181=AXIS2_PLACEMENT_3D('',#10906,#2457,#2458);
#2182=AXIS2_PLACEMENT_3D('',#10909,#2461,#2462);
#2183=AXIS2_PLACEMENT_3D('',#10913,#2464,#2465);
#2184=AXIS2_PLACEMENT_3D('',#10915,#2466,#2467);
#2185=AXIS2_PLACEMENT_3D('',#10918,#2469,#2470);
#2186=AXIS2_PLACEMENT_3D('',#10919,#2471,#2472);
#2187=AXIS2_PLACEMENT_3D('',#10923,#2475,#2476);
#2188=AXIS2_PLACEMENT_3D('',#10927,#2479,#2480);
#2189=AXIS2_PLACEMENT_3D('',#10929,#2481,#2482);
#2190=AXIS2_PLACEMENT_3D('',#10931,#2484,#2485);
#2191=AXIS2_PLACEMENT_3D('',#10933,#2486,#2487);
#2192=AXIS2_PLACEMENT_3D('',#10935,#2489,#2490);
#2193=AXIS2_PLACEMENT_3D('',#10936,#2491,#2492);
#2194=AXIS2_PLACEMENT_3D('',#10937,#2493,#2494);
#2347=DIRECTION('axis',(0.,0.,1.));
#2348=DIRECTION('refdir',(1.,0.,0.));
#2349=DIRECTION('center_axis',(0.,0.,-1.));
#2350=DIRECTION('ref_axis',(-0.707106781186547,-0.707106781186548,0.));
#2351=DIRECTION('center_axis',(0.,0.,1.));
#2352=DIRECTION('ref_axis',(-0.707106781186547,-0.707106781186548,0.));
#2353=DIRECTION('',(0.,0.,1.));
#2354=DIRECTION('center_axis',(0.,0.,-1.));
#2355=DIRECTION('ref_axis',(-0.707106781186547,-0.707106781186548,0.));
#2356=DIRECTION('',(0.,0.,-1.));
#2357=DIRECTION('center_axis',(0.,0.,-1.));
#2358=DIRECTION('ref_axis',(1.,0.,0.));
#2359=DIRECTION('',(0.,1.,0.));
#2360=DIRECTION('center_axis',(0.,0.,1.));
#2361=DIRECTION('ref_axis',(-0.707106781186548,0.707106781186547,0.));
#2362=DIRECTION('',(1.,0.,0.));
#2363=DIRECTION('',(0.,1.,0.));
#2364=DIRECTION('',(1.,0.,0.));
#2365=DIRECTION('center_axis',(0.,0.,-1.));
#2366=DIRECTION('ref_axis',(-0.707106781186548,0.707106781186547,0.));
#2367=DIRECTION('',(0.,0.,1.));
#2368=DIRECTION('center_axis',(0.,0.,-1.));
#2369=DIRECTION('ref_axis',(-0.707106781186548,0.707106781186547,0.));
#2370=DIRECTION('',(0.,0.,-1.));
#2371=DIRECTION('center_axis',(-1.,0.,0.));
#2372=DIRECTION('ref_axis',(0.,0.,-1.));
#2373=DIRECTION('',(0.,1.,0.));
#2374=DIRECTION('center_axis',(0.,0.,1.));
#2375=DIRECTION('ref_axis',(-1.,0.,0.));
#2376=DIRECTION('',(0.,1.,0.));
#2377=DIRECTION('',(-1.,0.,0.));
#2378=DIRECTION('',(-1.,0.,0.));
#2379=DIRECTION('',(0.,1.,0.));
#2380=DIRECTION('',(-1.,0.,0.));
#2381=DIRECTION('',(0.,-1.,0.));
#2382=DIRECTION('',(-1.,0.,0.));
#2383=DIRECTION('',(0.,-1.,0.));
#2384=DIRECTION('',(-1.,0.,0.));
#2385=DIRECTION('',(0.,-1.,0.));
#2386=DIRECTION('',(1.,0.,0.));
#2387=DIRECTION('center_axis',(1.,0.,0.));
#2388=DIRECTION('ref_axis',(0.,0.,1.));
#2389=DIRECTION('',(0.,0.,1.));
#2390=DIRECTION('',(0.,0.,1.));
#2391=DIRECTION('center_axis',(0.,1.,0.));
#2392=DIRECTION('ref_axis',(-1.,0.,0.));
#2393=DIRECTION('',(0.,0.,1.));
#2394=DIRECTION('',(0.86390887084174,0.,-0.503648153854405));
#2395=DIRECTION('center_axis',(1.,0.,0.));
#2396=DIRECTION('ref_axis',(0.,1.,0.));
#2397=DIRECTION('',(0.,1.,0.));
#2398=DIRECTION('',(0.,0.,1.));
#2399=DIRECTION('',(-1.20956479566685E-15,-1.,0.));
#2400=DIRECTION('center_axis',(0.,-1.,0.));
#2401=DIRECTION('ref_axis',(1.,0.,0.));
#2402=DIRECTION('',(-0.86390887084174,0.,0.503648153854405));
#2403=DIRECTION('',(0.,1.,0.));
#2404=DIRECTION('',(0.,1.,0.));
#2405=DIRECTION('',(0.,1.,0.));
#2406=DIRECTION('center_axis',(0.503648153854405,0.,0.86390887084174));
#2407=DIRECTION('ref_axis',(0.86390887084174,0.,-0.503648153854405));
#2408=DIRECTION('',(0.,1.,0.));
#2409=DIRECTION('',(0.86390887084174,0.,-0.503648153854405));
#2410=DIRECTION('center_axis',(0.,1.,0.));
#2411=DIRECTION('ref_axis',(-1.,0.,0.));
#2412=DIRECTION('',(0.,0.,1.));
#2413=DIRECTION('',(0.86390887084174,0.,-0.503648153854405));
#2414=DIRECTION('',(0.,1.,0.));
#2415=DIRECTION('',(0.,1.,0.));
#2416=DIRECTION('center_axis',(0.503648153854405,0.,0.86390887084174));
#2417=DIRECTION('ref_axis',(0.86390887084174,0.,-0.503648153854405));
#2418=DIRECTION('center_axis',(0.,1.,0.));
#2419=DIRECTION('ref_axis',(-1.,0.,0.));
#2420=DIRECTION('',(0.,0.,-1.));
#2421=DIRECTION('center_axis',(0.,1.,0.));
#2422=DIRECTION('ref_axis',(1.,0.,0.));
#2423=DIRECTION('',(0.,0.,1.));
#2424=DIRECTION('center_axis',(0.,1.,0.));
#2425=DIRECTION('ref_axis',(-1.00929365875014E-15,0.,1.));
#2426=DIRECTION('center_axis',(0.,1.,0.));
#2427=DIRECTION('ref_axis',(-1.,0.,4.84460956200068E-15));
#2428=DIRECTION('',(0.,0.,-1.));
#2429=DIRECTION('center_axis',(0.,-1.,0.));
#2430=DIRECTION('ref_axis',(1.,0.,0.));
#2431=DIRECTION('center_axis',(0.,1.,0.));
#2432=DIRECTION('ref_axis',(1.,0.,0.));
#2433=DIRECTION('',(0.,0.,-1.));
#2434=DIRECTION('',(0.,0.,1.));
#2435=DIRECTION('center_axis',(1.,0.,0.));
#2436=DIRECTION('ref_axis',(0.,0.,-1.));
#2437=DIRECTION('',(0.,-1.,0.));
#2438=DIRECTION('',(0.,0.,1.));
#2439=DIRECTION('center_axis',(0.,1.,0.));
#2440=DIRECTION('ref_axis',(1.,0.,0.));
#2441=DIRECTION('',(0.,0.,-1.));
#2442=DIRECTION('center_axis',(0.,1.,0.));
#2443=DIRECTION('ref_axis',(-1.,0.,4.84460956200068E-15));
#2444=DIRECTION('center_axis',(0.,1.,0.));
#2445=DIRECTION('ref_axis',(-1.00929365875014E-15,0.,1.));
#2446=DIRECTION('center_axis',(0.,-1.,0.));
#2447=DIRECTION('ref_axis',(1.,0.,0.));
#2448=DIRECTION('center_axis',(0.,1.,0.));
#2449=DIRECTION('ref_axis',(1.,0.,0.));
#2450=DIRECTION('',(0.,1.,0.));
#2451=DIRECTION('center_axis',(0.,1.,0.));
#2452=DIRECTION('ref_axis',(-1.,0.,4.84460956200068E-15));
#2453=DIRECTION('',(0.,1.,0.));
#2454=DIRECTION('center_axis',(0.,1.,0.));
#2455=DIRECTION('ref_axis',(-1.00929365875014E-15,0.,1.));
#2456=DIRECTION('',(0.,1.,0.));
#2457=DIRECTION('center_axis',(0.,1.,0.));
#2458=DIRECTION('ref_axis',(1.,0.,0.));
#2459=DIRECTION('',(0.,0.,-1.));
#2460=DIRECTION('',(0.,0.,1.));
#2461=DIRECTION('center_axis',(0.,1.,0.));
#2462=DIRECTION('ref_axis',(1.,0.,0.));
#2463=DIRECTION('',(0.,0.,1.));
#2464=DIRECTION('center_axis',(0.,1.,0.));
#2465=DIRECTION('ref_axis',(-1.,0.,4.84460956200068E-15));
#2466=DIRECTION('center_axis',(0.,1.,0.));
#2467=DIRECTION('ref_axis',(-1.00929365875014E-15,0.,1.));
#2468=DIRECTION('',(0.,0.,-1.));
#2469=DIRECTION('center_axis',(0.,-1.,0.));
#2470=DIRECTION('ref_axis',(1.,0.,0.));
#2471=DIRECTION('center_axis',(-1.,0.,0.));
#2472=DIRECTION('ref_axis',(0.,0.,1.));
#2473=DIRECTION('',(0.,1.,0.));
#2474=DIRECTION('',(0.,0.,1.));
#2475=DIRECTION('center_axis',(1.,0.,0.));
#2476=DIRECTION('ref_axis',(0.,0.,-1.));
#2477=DIRECTION('',(0.,0.,-1.));
#2478=DIRECTION('',(0.,-1.,0.));
#2479=DIRECTION('center_axis',(0.,1.,0.));
#2480=DIRECTION('ref_axis',(1.,0.,0.));
#2481=DIRECTION('center_axis',(0.,-1.,0.));
#2482=DIRECTION('ref_axis',(1.,0.,0.));
#2483=DIRECTION('',(0.,1.,0.));
#2484=DIRECTION('center_axis',(0.,1.,0.));
#2485=DIRECTION('ref_axis',(-1.,0.,4.84460956200068E-15));
#2486=DIRECTION('center_axis',(0.,1.,0.));
#2487=DIRECTION('ref_axis',(-1.,0.,4.84460956200068E-15));
#2488=DIRECTION('',(0.,1.,0.));
#2489=DIRECTION('center_axis',(0.,1.,0.));
#2490=DIRECTION('ref_axis',(-1.00929365875014E-15,0.,1.));
#2491=DIRECTION('center_axis',(0.,1.,0.));
#2492=DIRECTION('ref_axis',(-1.00929365875014E-15,0.,1.));
#2493=DIRECTION('center_axis',(0.,1.,0.));
#2494=DIRECTION('ref_axis',(1.,0.,0.));
#9786=CARTESIAN_POINT('',(0.,0.,0.));
#9787=CARTESIAN_POINT('Origin',(-33.8518529101985,-1.5,308.5));
#9788=CARTESIAN_POINT('',(-40.3518529101985,-1.5,307.));
#9789=CARTESIAN_POINT('',(-33.8518529101985,-8.,307.));
#9790=CARTESIAN_POINT('Origin',(-33.8518529101985,-1.5,307.));
#9791=CARTESIAN_POINT('',(-33.8518529101985,-8.,309.));
#9792=CARTESIAN_POINT('',(-33.8518529101985,-8.,308.5));
#9793=CARTESIAN_POINT('',(-40.3518529101985,-1.5,309.));
#9794=CARTESIAN_POINT('Origin',(-33.8518529101985,-1.5,309.));
#9795=CARTESIAN_POINT('',(-40.3518529101985,-1.5,308.5));
#9796=CARTESIAN_POINT('Origin',(-40.3518529101985,0.,307.));
#9797=CARTESIAN_POINT('',(-40.3518529101985,1.5,307.));
#9798=CARTESIAN_POINT('',(-40.3518529101985,0.,307.));
#9799=CARTESIAN_POINT('',(-33.8518529101985,8.,307.));
#9800=CARTESIAN_POINT('Origin',(-33.8518529101985,1.5,307.));
#9801=CARTESIAN_POINT('',(19.6481470898015,8.,307.));
#9802=CARTESIAN_POINT('',(19.6481470898015,8.,307.));
#9803=CARTESIAN_POINT('',(19.6481470898015,-8.,307.));
#9804=CARTESIAN_POINT('',(19.6481470898015,0.,307.));
#9805=CARTESIAN_POINT('',(19.6481470898015,-8.,307.));
#9806=CARTESIAN_POINT('Origin',(-33.8518529101985,1.5,308.5));
#9807=CARTESIAN_POINT('',(-40.3518529101985,1.5,309.));
#9808=CARTESIAN_POINT('',(-40.3518529101985,1.5,308.5));
#9809=CARTESIAN_POINT('',(-33.8518529101985,8.,309.));
#9810=CARTESIAN_POINT('Origin',(-33.8518529101985,1.5,309.));
#9811=CARTESIAN_POINT('',(-33.8518529101985,8.,308.5));
#9812=CARTESIAN_POINT('Origin',(-40.3518529101985,0.,309.));
#9813=CARTESIAN_POINT('',(-40.3518529101985,0.,309.));
#9814=CARTESIAN_POINT('Origin',(19.6481470898015,0.,309.));
#9815=CARTESIAN_POINT('',(-20.0405545273386,6.,309.));
#9816=CARTESIAN_POINT('',(-20.0405545273386,8.,309.));
#9817=CARTESIAN_POINT('',(-20.0405545273386,-8.,309.));
#9818=CARTESIAN_POINT('',(-40.3518529101985,8.,309.));
#9819=CARTESIAN_POINT('',(-20.0405545273386,-8.,309.));
#9820=CARTESIAN_POINT('',(-40.3518529101985,-8.,309.));
#9821=CARTESIAN_POINT('',(-20.0405545273386,-6.,309.));
#9822=CARTESIAN_POINT('',(-20.0405545273386,-8.,309.));
#9823=CARTESIAN_POINT('',(16.317900533139,-6.,309.));
#9824=CARTESIAN_POINT('',(-40.3518529101985,-6.,309.));
#9825=CARTESIAN_POINT('',(16.317900533139,-8.,309.));
#9826=CARTESIAN_POINT('',(16.317900533139,-8.,309.));
#9827=CARTESIAN_POINT('',(19.6481470898015,-8.,309.));
#9828=CARTESIAN_POINT('',(-40.3518529101985,-8.,309.));
#9829=CARTESIAN_POINT('',(19.6481470898015,8.,309.));
#9830=CARTESIAN_POINT('',(19.6481470898015,0.,309.));
#9831=CARTESIAN_POINT('',(16.317900533139,8.,309.));
#9832=CARTESIAN_POINT('',(-40.3518529101985,8.,309.));
#9833=CARTESIAN_POINT('',(16.317900533139,6.,309.));
#9834=CARTESIAN_POINT('',(16.317900533139,-8.,309.));
#9835=CARTESIAN_POINT('',(-40.3518529101985,6.,309.));
#9836=CARTESIAN_POINT('Origin',(19.6481470898015,0.,307.));
#9837=CARTESIAN_POINT('',(19.6481470898015,-8.,309.));
#9838=CARTESIAN_POINT('',(19.6481470898015,8.,309.));
#9839=CARTESIAN_POINT('Origin',(-16.022313954939,1.83573964553602,309.));
#9840=CARTESIAN_POINT('',(-16.022313954939,1.83573964553602,315.598323807971));
#9841=CARTESIAN_POINT('',(-34.7643786318829,1.83573964553602,326.55931644625));
#9842=CARTESIAN_POINT('Ctrl Pts',(-16.0223139548895,1.83573964553602,315.598323807965));
#9843=CARTESIAN_POINT('Ctrl Pts',(-16.6152689891987,1.83573964553602,315.668297772475));
#9844=CARTESIAN_POINT('Ctrl Pts',(-17.2033333974167,1.83573964553602,315.740204222438));
#9845=CARTESIAN_POINT('Ctrl Pts',(-17.7851093363551,1.83573964553602,315.814088969387));
#9846=CARTESIAN_POINT('Ctrl Pts',(-18.4542017359588,1.83573964553602,315.899062787177));
#9847=CARTESIAN_POINT('Ctrl Pts',(-19.1149750768524,1.83573964553602,315.986652476638));
#9848=CARTESIAN_POINT('Ctrl Pts',(-19.7652319532494,1.83573964553602,316.076948464976));
#9849=CARTESIAN_POINT('Ctrl Pts',(-20.4968760662518,1.83573964553602,316.178546050013));
#9850=CARTESIAN_POINT('Ctrl Pts',(-21.2152020044943,1.83573964553602,316.283568335362));
#9851=CARTESIAN_POINT('Ctrl Pts',(-21.9170421525721,1.83573964553602,316.392187427951));
#9852=CARTESIAN_POINT('Ctrl Pts',(-22.4830261868681,1.83573964553602,316.479780980975));
#9853=CARTESIAN_POINT('Ctrl Pts',(-23.0382867152506,1.83573964553602,316.569714291766));
#9854=CARTESIAN_POINT('Ctrl Pts',(-23.5811846866938,1.83573964553602,316.662104539026));
#9855=CARTESIAN_POINT('Ctrl Pts',(-24.0619814687136,1.83573964553602,316.743926420685));
#9856=CARTESIAN_POINT('Ctrl Pts',(-24.5330814352488,1.83573964553602,316.827675498925));
#9857=CARTESIAN_POINT('Ctrl Pts',(-24.9933830518898,1.83573964553602,316.913452048499));
#9858=CARTESIAN_POINT('Ctrl Pts',(-25.4232276652359,1.83573964553602,316.993552978959));
#9859=CARTESIAN_POINT('Ctrl Pts',(-25.8436552271082,1.83573964553602,317.07542204276));
#9860=CARTESIAN_POINT('Ctrl Pts',(-26.2538110895873,1.83573964553602,317.159156712438));
#9861=CARTESIAN_POINT('Ctrl Pts',(-26.6441668564352,1.83573964553602,317.238849127405));
#9862=CARTESIAN_POINT('Ctrl Pts',(-27.0252184159128,1.83573964553602,317.320231429346));
#9863=CARTESIAN_POINT('Ctrl Pts',(-27.3962737071739,1.83573964553602,317.403401459965));
#9864=CARTESIAN_POINT('Ctrl Pts',(-27.7503453005567,1.83573964553602,317.482764686839));
#9865=CARTESIAN_POINT('Ctrl Pts',(-28.0953145640723,1.83573964553602,317.563755774749));
#9866=CARTESIAN_POINT('Ctrl Pts',(-28.4306252622026,1.83573964553602,317.646471925112));
#9867=CARTESIAN_POINT('Ctrl Pts',(-28.7501141835393,1.83573964553602,317.725285079014));
#9868=CARTESIAN_POINT('Ctrl Pts',(-29.0608342542028,1.83573964553602,317.805664336882));
#9869=CARTESIAN_POINT('Ctrl Pts',(-29.3623498110856,1.83573964553602,317.887704925849));
#9870=CARTESIAN_POINT('Ctrl Pts',(-29.6523265222377,1.83573964553602,317.96660586355));
#9871=CARTESIAN_POINT('Ctrl Pts',(-29.9337895272155,1.83573964553602,318.047043401166));
#9872=CARTESIAN_POINT('Ctrl Pts',(-30.2063979120281,1.83573964553602,318.12911291368));
#9873=CARTESIAN_POINT('Ctrl Pts',(-30.4741983207634,1.83573964553602,318.209734971622));
#9874=CARTESIAN_POINT('Ctrl Pts',(-30.733453478094,1.83573964553602,318.291931941205));
#9875=CARTESIAN_POINT('Ctrl Pts',(-30.9838897802548,1.83573964553602,318.375804995173));
#9876=CARTESIAN_POINT('Ctrl Pts',(-31.235085850916,1.83573964553602,318.459932501487));
#9877=CARTESIAN_POINT('Ctrl Pts',(-31.4774094804883,1.83573964553602,318.545746357418));
#9878=CARTESIAN_POINT('Ctrl Pts',(-31.7106360658033,1.83573964553602,318.633358865222));
#9879=CARTESIAN_POINT('Ctrl Pts',(-31.9446281429948,1.83573964553602,318.721258933138));
#9880=CARTESIAN_POINT('Ctrl Pts',(-32.1694633663929,1.83573964553602,318.810969561697));
#9881=CARTESIAN_POINT('Ctrl Pts',(-32.3849665985943,1.83573964553602,318.902613194341));
#9882=CARTESIAN_POINT('Ctrl Pts',(-32.6034685743786,1.83573964553602,318.995532054982));
#9883=CARTESIAN_POINT('Ctrl Pts',(-32.8123770460666,1.83573964553602,319.090438190617));
#9884=CARTESIAN_POINT('Ctrl Pts',(-33.0115629265537,1.83573964553602,319.187467234392));
#9885=CARTESIAN_POINT('Ctrl Pts',(-33.2245143369608,1.83573964553602,319.291201854897));
#9886=CARTESIAN_POINT('Ctrl Pts',(-33.4263528949916,1.83573964553602,319.397363178007));
#9887=CARTESIAN_POINT('Ctrl Pts',(-33.6169817448998,1.83573964553602,319.506123424921));
#9888=CARTESIAN_POINT('Ctrl Pts',(-33.8180636092573,1.83573964553602,319.620847472347));
#9889=CARTESIAN_POINT('Ctrl Pts',(-34.0066730565997,1.83573964553602,319.738463663551));
#9890=CARTESIAN_POINT('Ctrl Pts',(-34.1827589496644,1.83573964553602,319.859176194319));
#9891=CARTESIAN_POINT('Ctrl Pts',(-34.3681788381234,1.83573964553602,319.986287478482));
#9892=CARTESIAN_POINT('Ctrl Pts',(-34.5397127794776,1.83573964553602,320.116832623688));
#9893=CARTESIAN_POINT('Ctrl Pts',(-34.6973613341441,1.83573964553602,320.251044787742));
#9894=CARTESIAN_POINT('Ctrl Pts',(-34.8627482473033,1.83573964553602,320.391844908417));
#9895=CARTESIAN_POINT('Ctrl Pts',(-35.0128537576466,1.83573964553602,320.536681652576));
#9896=CARTESIAN_POINT('Ctrl Pts',(-35.1477349540007,1.83573964553602,320.685808129403));
#9897=CARTESIAN_POINT('Ctrl Pts',(-35.2876536117633,1.83573964553602,320.840504091765));
#9898=CARTESIAN_POINT('Ctrl Pts',(-35.4111905301923,1.83573964553602,320.999817147191));
#9899=CARTESIAN_POINT('Ctrl Pts',(-35.5184561722676,1.83573964553602,321.163999379985));
#9900=CARTESIAN_POINT('Ctrl Pts',(-35.6268225696939,1.83573964553602,321.329866443708));
#9901=CARTESIAN_POINT('Ctrl Pts',(-35.7185833239258,1.83573964553602,321.500703866045));
#9902=CARTESIAN_POINT('Ctrl Pts',(-35.7938813306046,1.83573964553602,321.676728264262));
#9903=CARTESIAN_POINT('Ctrl Pts',(-35.8676199592198,1.83573964553602,321.849107299244));
#9904=CARTESIAN_POINT('Ctrl Pts',(-35.9255719424798,1.83573964553602,322.026461132262));
#9905=CARTESIAN_POINT('Ctrl Pts',(-35.9678797220083,1.83573964553602,322.208943590835));
#9906=CARTESIAN_POINT('Ctrl Pts',(-36.0118309030396,1.83573964553602,322.398514389896));
#9907=CARTESIAN_POINT('Ctrl Pts',(-36.0388994930129,1.83573964553602,322.593619826998));
#9908=CARTESIAN_POINT('Ctrl Pts',(-36.0492380796555,1.83573964553602,322.794372875513));
#9909=CARTESIAN_POINT('Ctrl Pts',(-36.0601918922669,1.83573964553602,323.007072285077));
#9910=CARTESIAN_POINT('Ctrl Pts',(-36.0523658257608,1.83573964553602,323.22611083602));
#9911=CARTESIAN_POINT('Ctrl Pts',(-36.0259258665584,1.83573964553602,323.451564467522));
#9912=CARTESIAN_POINT('Ctrl Pts',(-35.9978345161503,1.83573964553602,323.691099518042));
#9913=CARTESIAN_POINT('Ctrl Pts',(-35.9487323336772,1.83573964553602,323.937875220018));
#9914=CARTESIAN_POINT('Ctrl Pts',(-35.8787910094436,1.83573964553602,324.191930695693));
#9915=CARTESIAN_POINT('Ctrl Pts',(-35.8085289173363,1.83573964553602,324.447151331388));
#9916=CARTESIAN_POINT('Ctrl Pts',(-35.7172368742329,1.83573964553602,324.709717470243));
#9917=CARTESIAN_POINT('Ctrl Pts',(-35.6050496765245,1.83573964553602,324.979633431004));
#9918=CARTESIAN_POINT('Ctrl Pts',(-35.4952270641624,1.83573964553602,325.243860335095));
#9919=CARTESIAN_POINT('Ctrl Pts',(-35.3653812147248,1.83573964553602,325.515129206621));
#9920=CARTESIAN_POINT('Ctrl Pts',(-35.2155923657828,1.83573964553602,325.793428673214));
#9921=CARTESIAN_POINT('Ctrl Pts',(-35.0812280121379,1.83573964553602,326.043070273457));
#9922=CARTESIAN_POINT('Ctrl Pts',(-34.930816038242,1.83573964553602,326.298368234338));
#9923=CARTESIAN_POINT('Ctrl Pts',(-34.764378631884,1.83573964553602,326.559316446249));
#9924=CARTESIAN_POINT('',(-16.0223147731638,1.83573964553602,317.612324242706));
#9925=CARTESIAN_POINT('',(-16.022313954939,1.83573964553602,309.));
#9926=CARTESIAN_POINT('',(-33.0349479481876,1.83573964553602,325.551079813359));
#9927=CARTESIAN_POINT('Ctrl Pts',(-33.0349479481876,1.83573964553602,325.551079813359));
#9928=CARTESIAN_POINT('Ctrl Pts',(-33.0661229600418,1.83573964553602,325.502919119248));
#9929=CARTESIAN_POINT('Ctrl Pts',(-33.0982940340322,1.83573964553602,325.452411922573));
#9930=CARTESIAN_POINT('Ctrl Pts',(-33.131233956743,1.83573964553602,325.399647814597));
#9931=CARTESIAN_POINT('Ctrl Pts',(-33.1635771509031,1.83573964553602,325.347839563438));
#9932=CARTESIAN_POINT('Ctrl Pts',(-33.1966614942152,1.83573964553602,325.293855191547));
#9933=CARTESIAN_POINT('Ctrl Pts',(-33.2302370146661,1.83573964553602,325.237815505789));
#9934=CARTESIAN_POINT('Ctrl Pts',(-33.2631969912884,1.83573964553601,325.182803201953));
#9935=CARTESIAN_POINT('Ctrl Pts',(-33.2966301760354,1.83573964553601,325.125810009937));
#9936=CARTESIAN_POINT('Ctrl Pts',(-33.3302677882625,1.83573964553601,325.066988767008));
#9937=CARTESIAN_POINT('Ctrl Pts',(-33.3645508807256,1.83573964553601,325.007038789092));
#9938=CARTESIAN_POINT('Ctrl Pts',(-33.3990463607999,1.835739645536,324.945189352181));
#9939=CARTESIAN_POINT('Ctrl Pts',(-33.4334361488523,1.835739645536,324.881649213761));
#9940=CARTESIAN_POINT('Ctrl Pts',(-33.4655449686488,1.83573964553599,324.822323496158));
#9941=CARTESIAN_POINT('Ctrl Pts',(-33.4975612585259,1.83573964553599,324.761524029569));
#9942=CARTESIAN_POINT('Ctrl Pts',(-33.5292005359126,1.83573964553599,324.699463434241));
#9943=CARTESIAN_POINT('Ctrl Pts',(-33.5602287107319,1.83573964553599,324.638601519549));
#9944=CARTESIAN_POINT('Ctrl Pts',(-33.5908941148617,1.83573964553599,324.576526494744));
#9945=CARTESIAN_POINT('Ctrl Pts',(-33.6209067634036,1.83573964553598,324.513482761705));
#9946=CARTESIAN_POINT('Ctrl Pts',(-33.6503193146855,1.83573964553598,324.451699576245));
#9947=CARTESIAN_POINT('Ctrl Pts',(-33.6791047579574,1.83573964553598,324.38898581439));
#9948=CARTESIAN_POINT('Ctrl Pts',(-33.7069719015286,1.83573964553598,324.325617311444));
#9949=CARTESIAN_POINT('Ctrl Pts',(-33.7342650960075,1.83573964553598,324.26355394028));
#9950=CARTESIAN_POINT('Ctrl Pts',(-33.7606772237622,1.83573964553597,324.200862311328));
#9951=CARTESIAN_POINT('Ctrl Pts',(-33.7859199496834,1.83573964553597,324.137849069499));
#9952=CARTESIAN_POINT('Ctrl Pts',(-33.810150966544,1.83573964553597,324.077361349989));
#9953=CARTESIAN_POINT('Ctrl Pts',(-33.8333042102568,1.83573964553597,324.016577250446));
#9954=CARTESIAN_POINT('Ctrl Pts',(-33.855114095281,1.83573964553597,323.95581369679));
#9955=CARTESIAN_POINT('Ctrl Pts',(-33.8714715090491,1.83573964553597,323.910241031548));
#9956=CARTESIAN_POINT('Ctrl Pts',(-33.8870730522591,1.83573964553596,323.864680805165));
#9957=CARTESIAN_POINT('Ctrl Pts',(-33.9018036987318,1.83573964553596,323.81928501815));
#9958=CARTESIAN_POINT('Ctrl Pts',(-33.903388516175,1.83573964553596,323.814401048173));
#9959=CARTESIAN_POINT('Ctrl Pts',(-33.9049632511178,1.83573964553596,323.809518997366));
#9960=CARTESIAN_POINT('Ctrl Pts',(-33.9065277589274,1.83573964553596,323.804639066578));
#9961=CARTESIAN_POINT('Ctrl Pts',(-33.9081860973494,1.83573964553596,323.79946646426));
#9962=CARTESIAN_POINT('Ctrl Pts',(-33.9098356620974,1.83573964553597,323.794287785025));
#9963=CARTESIAN_POINT('Ctrl Pts',(-33.9114772546065,1.83573964553597,323.78909981003));
#9964=CARTESIAN_POINT('Ctrl Pts',(-33.9220168706031,1.83573964553597,323.755791139372));
#9965=CARTESIAN_POINT('Ctrl Pts',(-33.9322172469864,1.83573964553596,323.722136686936));
#9966=CARTESIAN_POINT('Ctrl Pts',(-33.9420163332251,1.83573964553596,323.688108868225));
#9967=CARTESIAN_POINT('Ctrl Pts',(-33.9515815869685,1.83573964553596,323.654893044588));
#9968=CARTESIAN_POINT('Ctrl Pts',(-33.9607644832687,1.83573964553596,323.621321202823));
#9969=CARTESIAN_POINT('Ctrl Pts',(-33.9694792291379,1.83573964553596,323.587406806218));
#9970=CARTESIAN_POINT('Ctrl Pts',(-33.9778537831925,1.83573964553596,323.554816303654));
#9971=CARTESIAN_POINT('Ctrl Pts',(-33.9857959509883,1.83573964553596,323.521909316756));
#9972=CARTESIAN_POINT('Ctrl Pts',(-33.9932039201841,1.83573964553596,323.488737145608));
#9973=CARTESIAN_POINT('Ctrl Pts',(-34.0001578485148,1.83573964553596,323.457598125635));
#9974=CARTESIAN_POINT('Ctrl Pts',(-34.0066408917444,1.83573964553596,323.426225452903));
#9975=CARTESIAN_POINT('Ctrl Pts',(-34.0125475629435,1.83573964553596,323.394697592393));
#9976=CARTESIAN_POINT('Ctrl Pts',(-34.0204218787242,1.83573964553596,323.352667094813));
#9977=CARTESIAN_POINT('Ctrl Pts',(-34.0276034892945,1.83573964553596,323.310601967879));
#9978=CARTESIAN_POINT('Ctrl Pts',(-34.0338763811083,1.83573964553596,323.268600643377));
#9979=CARTESIAN_POINT('Ctrl Pts',(-34.0402272820105,1.83573964553596,323.226076994381));
#9980=CARTESIAN_POINT('Ctrl Pts',(-34.0456467538288,1.83573964553595,323.183620856352));
#9981=CARTESIAN_POINT('Ctrl Pts',(-34.0498606505411,1.83573964553595,323.141342035231));
#9982=CARTESIAN_POINT('Ctrl Pts',(-34.0535478101644,1.83573964553595,323.10434806675));
#9983=CARTESIAN_POINT('Ctrl Pts',(-34.0563110736814,1.83573964553595,323.067491370795));
#9984=CARTESIAN_POINT('Ctrl Pts',(-34.0579366305321,1.83573964553595,323.030826699035));
#9985=CARTESIAN_POINT('Ctrl Pts',(-34.0586478116543,1.83573964553595,323.01478590514));
#9986=CARTESIAN_POINT('Ctrl Pts',(-34.0591408787633,1.83573964553595,322.998781480843));
#9987=CARTESIAN_POINT('Ctrl Pts',(-34.0593963692177,1.83573964553595,322.982815529254));
#9988=CARTESIAN_POINT('Ctrl Pts',(-34.0595457502028,1.83573964553595,322.973480505046));
#9989=CARTESIAN_POINT('Ctrl Pts',(-34.059613897403,1.83573964553595,322.964158598581));
#9990=CARTESIAN_POINT('Ctrl Pts',(-34.0595967827887,1.83573964553595,322.954849884516));
#9991=CARTESIAN_POINT('Ctrl Pts',(-34.0595895490535,1.83573964553595,322.950915424108));
#9992=CARTESIAN_POINT('Ctrl Pts',(-34.0595670825154,1.83573964553595,322.946983316998));
#9993=CARTESIAN_POINT('Ctrl Pts',(-34.0595290738543,1.83573964553595,322.943053552826));
#9994=CARTESIAN_POINT('Ctrl Pts',(-34.0594966483836,1.83573964553595,322.939701041856));
#9995=CARTESIAN_POINT('Ctrl Pts',(-34.0594528840535,1.83573964553596,322.936350674456));
#9996=CARTESIAN_POINT('Ctrl Pts',(-34.0593979182879,1.83573964553596,322.933016227715));
#9997=CARTESIAN_POINT('Ctrl Pts',(-34.0588959733313,1.83573964553596,322.902566206589));
#9998=CARTESIAN_POINT('Ctrl Pts',(-34.0574546420989,1.83573964553595,322.873152102209));
#9999=CARTESIAN_POINT('Ctrl Pts',(-34.0551137779108,1.83573964553596,322.844741632322));
#10000=CARTESIAN_POINT('Ctrl Pts',(-34.0525864883566,1.83573964553596,322.814068565452));
#10001=CARTESIAN_POINT('Ctrl Pts',(-34.0490105210139,1.83573964553596,322.784564394402));
#10002=CARTESIAN_POINT('Ctrl Pts',(-34.0444803381258,1.83573964553597,322.756139919022));
#10003=CARTESIAN_POINT('Ctrl Pts',(-34.0395034099273,1.83573964553598,322.724912355691));
#10004=CARTESIAN_POINT('Ctrl Pts',(-34.033374665099,1.83573964553598,322.694985969688));
#10005=CARTESIAN_POINT('Ctrl Pts',(-34.0262736095825,1.83573964553599,322.66620941123));
#10006=CARTESIAN_POINT('Ctrl Pts',(-34.0190897812723,1.835739645536,322.637097421492));
#10007=CARTESIAN_POINT('Ctrl Pts',(-34.0109116401738,1.83573964553601,322.609159473663));
#10008=CARTESIAN_POINT('Ctrl Pts',(-34.0019715940061,1.83573964553601,322.582244612095));
#10009=CARTESIAN_POINT('Ctrl Pts',(-33.9936074678832,1.83573964553602,322.557063612745));
#10010=CARTESIAN_POINT('Ctrl Pts',(-33.9845774637373,1.83573964553602,322.532776674166));
#10011=CARTESIAN_POINT('Ctrl Pts',(-33.9750984607969,1.83573964553602,322.509294674303));
#10012=CARTESIAN_POINT('Ctrl Pts',(-33.9715914785727,1.83573964553602,322.500606950854));
#10013=CARTESIAN_POINT('Ctrl Pts',(-33.9680232387229,1.83573964553602,322.492029864451));
#10014=CARTESIAN_POINT('Ctrl Pts',(-33.9644053373266,1.83573964553602,322.483560715069));
#10015=CARTESIAN_POINT('Ctrl Pts',(-33.9616919112793,1.83573964553602,322.477208853033));
#10016=CARTESIAN_POINT('Ctrl Pts',(-33.9589505570832,1.83573964553602,322.470917726621));
#10017=CARTESIAN_POINT('Ctrl Pts',(-33.9561862549531,1.83573964553602,322.464686624446));
#10018=CARTESIAN_POINT('Ctrl Pts',(-33.9554525044853,1.83573964553602,322.46303265396));
#10019=CARTESIAN_POINT('Ctrl Pts',(-33.9547180544517,1.83573964553602,322.461384960683));
#10020=CARTESIAN_POINT('Ctrl Pts',(-33.9539800208225,1.83573964553602,322.459736890762));
#10021=CARTESIAN_POINT('Ctrl Pts',(-33.9463767394291,1.83573964553602,322.442758342803));
#10022=CARTESIAN_POINT('Ctrl Pts',(-33.9381513961156,1.83573964553602,322.425207535287));
#10023=CARTESIAN_POINT('Ctrl Pts',(-33.9292861005445,1.83573964553602,322.407067430352));
#10024=CARTESIAN_POINT('Ctrl Pts',(-33.9163337908113,1.83573964553602,322.380564506018));
#10025=CARTESIAN_POINT('Ctrl Pts',(-33.901311364989,1.83573964553602,322.352146899478));
#10026=CARTESIAN_POINT('Ctrl Pts',(-33.8837148715601,1.83573964553602,322.321871781303));
#10027=CARTESIAN_POINT('Ctrl Pts',(-33.8661649416896,1.83573964553602,322.291676776661));
#10028=CARTESIAN_POINT('Ctrl Pts',(-33.8460516650248,1.83573964553602,322.259633661156));
#10029=CARTESIAN_POINT('Ctrl Pts',(-33.8228757301491,1.83573964553602,322.225850752003));
#10030=CARTESIAN_POINT('Ctrl Pts',(-33.8025967871328,1.83573964553602,322.196290706493));
#10031=CARTESIAN_POINT('Ctrl Pts',(-33.779971552621,1.83573964553602,322.165399323574));
#10032=CARTESIAN_POINT('Ctrl Pts',(-33.754694371687,1.83573964553602,322.133284613885));
#10033=CARTESIAN_POINT('Ctrl Pts',(-33.7324716601145,1.83573964553602,322.105050613722));
#10034=CARTESIAN_POINT('Ctrl Pts',(-33.7081987854865,1.83573964553602,322.075871552253));
#10035=CARTESIAN_POINT('Ctrl Pts',(-33.681702675014,1.83573964553602,322.045842732977));
#10036=CARTESIAN_POINT('Ctrl Pts',(-33.6586439822492,1.83573964553602,322.019709640027));
#10037=CARTESIAN_POINT('Ctrl Pts',(-33.6339015919019,1.83573964553602,321.992933294462));
#10038=CARTESIAN_POINT('Ctrl Pts',(-33.6073906529172,1.83573964553602,321.965589170075));
#10039=CARTESIAN_POINT('Ctrl Pts',(-33.5957921171115,1.83573964553602,321.953626115656));
#10040=CARTESIAN_POINT('Ctrl Pts',(-33.5838554703109,1.83573964553602,321.941554535908));
#10041=CARTESIAN_POINT('Ctrl Pts',(-33.5715756391018,1.83573964553602,321.929381449567));
#10042=CARTESIAN_POINT('Ctrl Pts',(-33.5675028306389,1.83573964553602,321.925344044799));
#10043=CARTESIAN_POINT('Ctrl Pts',(-33.5633922819587,1.83573964553602,321.921295477467));
#10044=CARTESIAN_POINT('Ctrl Pts',(-33.5592438414042,1.83573964553602,321.917236013815));
#10045=CARTESIAN_POINT('Ctrl Pts',(-33.5566208888724,1.83573964553602,321.914669319097));
#10046=CARTESIAN_POINT('Ctrl Pts',(-33.5539896374706,1.83573964553602,321.912104970658));
#10047=CARTESIAN_POINT('Ctrl Pts',(-33.5513503112792,1.83573964553602,321.90954312463));
#10048=CARTESIAN_POINT('Ctrl Pts',(-33.5083180543833,1.83573964553602,321.867774124349));
#10049=CARTESIAN_POINT('Ctrl Pts',(-33.463127010343,1.83573964553602,321.826664476558));
#10050=CARTESIAN_POINT('Ctrl Pts',(-33.4162725739017,1.83573964553602,321.786383286682));
#10051=CARTESIAN_POINT('Ctrl Pts',(-33.3665511889838,1.83573964553602,321.743637354837));
#10052=CARTESIAN_POINT('Ctrl Pts',(-33.3149589484907,1.83573964553602,321.701824351088));
#10053=CARTESIAN_POINT('Ctrl Pts',(-33.2620971297531,1.83573964553602,321.661092478806));
#10054=CARTESIAN_POINT('Ctrl Pts',(-33.2081082235734,1.83573964553602,321.619492146397));
#10055=CARTESIAN_POINT('Ctrl Pts',(-33.1527972067788,1.83573964553602,321.579019172729));
#10056=CARTESIAN_POINT('Ctrl Pts',(-33.0967785132887,1.83573964553602,321.539780381638));
#10057=CARTESIAN_POINT('Ctrl Pts',(-33.045742165131,1.83573964553602,321.50403151856));
#10058=CARTESIAN_POINT('Ctrl Pts',(-32.9941189005934,1.83573964553602,321.469306192837));
#10059=CARTESIAN_POINT('Ctrl Pts',(-32.9423350670271,1.83573964553602,321.435653391126));
#10060=CARTESIAN_POINT('Ctrl Pts',(-32.9372797495765,1.83573964553602,321.432368087895));
#10061=CARTESIAN_POINT('Ctrl Pts',(-32.9322228666748,1.83573964553602,321.429092984523));
#10062=CARTESIAN_POINT('Ctrl Pts',(-32.9271647914283,1.83573964553602,321.425828112808));
#10063=CARTESIAN_POINT('Ctrl Pts',(-32.8846896414527,1.83573964553602,321.398411376407));
#10064=CARTESIAN_POINT('Ctrl Pts',(-32.842219263063,1.83573964553602,321.371890527538));
#10065=CARTESIAN_POINT('Ctrl Pts',(-32.8000105131935,1.83573964553602,321.346250280345));
#10066=CARTESIAN_POINT('Ctrl Pts',(-32.7565769533191,1.83573964553602,321.319866006585));
#10067=CARTESIAN_POINT('Ctrl Pts',(-32.7134202611095,1.83573964553602,321.2944140929));
#10068=CARTESIAN_POINT('Ctrl Pts',(-32.670764292969,1.83573964553602,321.269868505081));
#10069=CARTESIAN_POINT('Ctrl Pts',(-32.6268132809282,1.83573964553602,321.244577708205));
#10070=CARTESIAN_POINT('Ctrl Pts',(-32.5833936843695,1.83573964553602,321.220249017716));
#10071=CARTESIAN_POINT('Ctrl Pts',(-32.5406943694291,1.83573964553602,321.196845515525));
#10072=CARTESIAN_POINT('Ctrl Pts',(-32.4966341481514,1.83573964553602,321.172696100325));
#10073=CARTESIAN_POINT('Ctrl Pts',(-32.4533406689138,1.83573964553602,321.149531703507));
#10074=CARTESIAN_POINT('Ctrl Pts',(-32.4109654673342,1.83573964553602,321.127304250182));
#10075=CARTESIAN_POINT('Ctrl Pts',(-32.3671672942411,1.83573964553602,321.10433039255));
#10076=CARTESIAN_POINT('Ctrl Pts',(-32.324349910069,1.83573964553602,321.082357379127));
#10077=CARTESIAN_POINT('Ctrl Pts',(-32.2826247223161,1.83573964553602,321.061325523161));
#10078=CARTESIAN_POINT('Ctrl Pts',(-32.2560473384883,1.83573964553602,321.047929017629));
#10079=CARTESIAN_POINT('Ctrl Pts',(-32.2299119673399,1.83573964553602,321.034914232251));
#10080=CARTESIAN_POINT('Ctrl Pts',(-32.204236776274,1.83573964553602,321.022264635838));
#10081=CARTESIAN_POINT('Ctrl Pts',(-32.1918003556014,1.83573964553602,321.016137487575));
#10082=CARTESIAN_POINT('Ctrl Pts',(-32.1794717848192,1.83573964553602,321.010096008134));
#10083=CARTESIAN_POINT('Ctrl Pts',(-32.1672524930891,1.83573964553602,321.00413825892));
#10084=CARTESIAN_POINT('Ctrl Pts',(-32.1607841646539,1.83573964553602,321.000984501771));
#10085=CARTESIAN_POINT('Ctrl Pts',(-32.1543464511367,1.83573964553602,320.997854206509));
#10086=CARTESIAN_POINT('Ctrl Pts',(-32.147939519909,1.83573964553602,320.994747081604));
#10087=CARTESIAN_POINT('Ctrl Pts',(-32.1449378300415,1.83573964553602,320.993291372932));
#10088=CARTESIAN_POINT('Ctrl Pts',(-32.1419442747369,1.83573964553602,320.991841416804));
#10089=CARTESIAN_POINT('Ctrl Pts',(-32.1389545705401,1.83573964553602,320.990395103825));
#10090=CARTESIAN_POINT('Ctrl Pts',(-32.0264733109678,1.83573964553602,320.935980655161));
#10091=CARTESIAN_POINT('Ctrl Pts',(-31.908137444516,1.83573964553602,320.881253703151));
#10092=CARTESIAN_POINT('Ctrl Pts',(-31.7837893774404,1.83573964553602,320.826251984166));
#10093=CARTESIAN_POINT('Ctrl Pts',(-31.6585403111675,1.83573964553602,320.770851734623));
#10094=CARTESIAN_POINT('Ctrl Pts',(-31.5271915179057,1.83573964553602,320.715172504509));
#10095=CARTESIAN_POINT('Ctrl Pts',(-31.3895291454136,1.83573964553602,320.659258824958));
#10096=CARTESIAN_POINT('Ctrl Pts',(-31.2510604150361,1.83573964553602,320.60301763081));
#10097=CARTESIAN_POINT('Ctrl Pts',(-31.1062038344124,1.83573964553602,320.546538993237));
#10098=CARTESIAN_POINT('Ctrl Pts',(-30.9546898749326,1.83573964553602,320.489877692076));
#10099=CARTESIAN_POINT('Ctrl Pts',(-30.8022990163583,1.83573964553602,320.432888459126));
#10100=CARTESIAN_POINT('Ctrl Pts',(-30.6431734062554,1.83573964553602,320.375714174219));
#10101=CARTESIAN_POINT('Ctrl Pts',(-30.4769878213684,1.83573964553602,320.318423942592));
#10102=CARTESIAN_POINT('Ctrl Pts',(-30.3105628359861,1.83573964553602,320.261051180884));
#10103=CARTESIAN_POINT('Ctrl Pts',(-30.1370573939087,1.83573964553602,320.203561852257));
#10104=CARTESIAN_POINT('Ctrl Pts',(-29.9560955534919,1.83573964553602,320.146042878496));
#10105=CARTESIAN_POINT('Ctrl Pts',(-29.7752986487112,1.83573964553602,320.088576329758));
#10106=CARTESIAN_POINT('Ctrl Pts',(-29.5870587823504,1.83573964553602,320.031079883726));
#10107=CARTESIAN_POINT('Ctrl Pts',(-29.3909539457544,1.83573964553602,319.973662122803));
#10108=CARTESIAN_POINT('Ctrl Pts',(-29.2776290644937,1.83573964553602,319.940481600325));
#10109=CARTESIAN_POINT('Ctrl Pts',(-29.1616768600902,1.83573964553602,319.907327782954));
#10110=CARTESIAN_POINT('Ctrl Pts',(-29.043009016516,1.83573964553602,319.874225600227));
#10111=CARTESIAN_POINT('Ctrl Pts',(-28.8007656894285,1.83573964553602,319.80665225739));
#10112=CARTESIAN_POINT('Ctrl Pts',(-28.5473824685975,1.83573964553602,319.739066503176));
#10113=CARTESIAN_POINT('Ctrl Pts',(-28.2822169710412,1.83573964553602,319.671421318884));
#10114=CARTESIAN_POINT('Ctrl Pts',(-27.9983427087817,1.83573964553602,319.599003425291));
#10115=CARTESIAN_POINT('Ctrl Pts',(-27.700964380257,1.83573964553602,319.526517177977));
#10116=CARTESIAN_POINT('Ctrl Pts',(-27.3892358081502,1.83573964553602,319.453922151971));
#10117=CARTESIAN_POINT('Ctrl Pts',(-27.0354358203731,1.83573964553602,319.371529578393));
#10118=CARTESIAN_POINT('Ctrl Pts',(-26.663149516191,1.83573964553602,319.288996201745));
#10119=CARTESIAN_POINT('Ctrl Pts',(-26.271080031633,1.83573964553602,319.206292236006));
#10120=CARTESIAN_POINT('Ctrl Pts',(-25.8610062347746,1.83573964553602,319.119790402576));
#10121=CARTESIAN_POINT('Ctrl Pts',(-25.429286642215,1.83573964553602,319.033101515975));
#10122=CARTESIAN_POINT('Ctrl Pts',(-24.9744178788053,1.83573964553602,318.946230143728));
#10123=CARTESIAN_POINT('Ctrl Pts',(-24.6003130682804,1.83573964553602,318.874783166338));
#10124=CARTESIAN_POINT('Ctrl Pts',(-24.2105479126315,1.83573964553602,318.803213426619));
#10125=CARTESIAN_POINT('Ctrl Pts',(-23.8043103135764,1.83573964553602,318.731544709485));
#10126=CARTESIAN_POINT('Ctrl Pts',(-23.4432514353454,1.83573964553602,318.667846453407));
#10127=CARTESIAN_POINT('Ctrl Pts',(-23.0691794360944,1.83573964553602,318.604070244179));
#10128=CARTESIAN_POINT('Ctrl Pts',(-22.6815611843081,1.83573964553602,318.540246192317));
#10129=CARTESIAN_POINT('Ctrl Pts',(-22.3248548638107,1.83573964553602,318.481512005797));
#10130=CARTESIAN_POINT('Ctrl Pts',(-21.9566761681602,1.83573964553602,318.422737416197));
#10131=CARTESIAN_POINT('Ctrl Pts',(-21.5766520973531,1.83573964553602,318.363955779299));
#10132=CARTESIAN_POINT('Ctrl Pts',(-21.2206131023023,1.83573964553602,318.308884123221));
#10133=CARTESIAN_POINT('Ctrl Pts',(-20.8541763488,1.83573964553602,318.253806348451));
#10134=CARTESIAN_POINT('Ctrl Pts',(-20.477080807384,1.83573964553602,318.198757752451));
#10135=CARTESIAN_POINT('Ctrl Pts',(-20.1284259143964,1.83573964553602,318.147860936553));
#10136=CARTESIAN_POINT('Ctrl Pts',(-19.7706592399563,1.83573964553602,318.096989131011));
#10137=CARTESIAN_POINT('Ctrl Pts',(-19.4036184737005,1.83573964553602,318.046176242108));
#10138=CARTESIAN_POINT('Ctrl Pts',(-19.0501707445755,1.83573964553602,317.99724516457));
#10139=CARTESIAN_POINT('Ctrl Pts',(-18.6881227696217,1.83573964553602,317.948368742741));
#10140=CARTESIAN_POINT('Ctrl Pts',(-18.3173759377902,1.83573964553602,317.899582486812));
#10141=CARTESIAN_POINT('Ctrl Pts',(-17.9656988419601,1.83573964553602,317.853305601002));
#10142=CARTESIAN_POINT('Ctrl Pts',(-17.6061945905643,1.83573964553602,317.807109874995));
#10143=CARTESIAN_POINT('Ctrl Pts',(-17.238824839512,1.83573964553602,317.761030019511));
#10144=CARTESIAN_POINT('Ctrl Pts',(-16.9638795440795,1.83573964553602,317.726543131456));
#10145=CARTESIAN_POINT('Ctrl Pts',(-16.684529436466,1.83573964553602,317.692121232857));
#10146=CARTESIAN_POINT('Ctrl Pts',(-16.4007776292659,1.83573964553602,317.65778048784));
#10147=CARTESIAN_POINT('Ctrl Pts',(-16.2754547949549,1.83573964553602,317.642613432023));
#10148=CARTESIAN_POINT('Ctrl Pts',(-16.1493020013402,1.83573964553602,317.627460892713));
#10149=CARTESIAN_POINT('Ctrl Pts',(-16.0223151822762,1.83573964553602,317.612324258224));
#10150=CARTESIAN_POINT('',(-23.9503331469548,1.83573964553602,320.25486209));
#10151=CARTESIAN_POINT('Origin',(-16.022313954939,-1.83573964553602,309.));
#10152=CARTESIAN_POINT('',(-16.022313954939,-1.83573964553602,315.598323807971));
#10153=CARTESIAN_POINT('',(-16.022313954939,-1.83573964553602,315.598323807971));
#10154=CARTESIAN_POINT('',(-16.0223147731638,-1.83573964553602,317.612324242706));
#10155=CARTESIAN_POINT('',(-16.022313954939,-1.83573964553602,309.));
#10156=CARTESIAN_POINT('',(-16.0223151822762,1.83573964553602,317.612324258224));
#10157=CARTESIAN_POINT('Origin',(-40.3518529101985,-1.83573964553602,309.));
#10158=CARTESIAN_POINT('',(-34.7643786318829,-1.83573964553602,326.55931644625));
#10159=CARTESIAN_POINT('Ctrl Pts',(-34.764378631884,-1.83573964553602,326.559316446249));
#10160=CARTESIAN_POINT('Ctrl Pts',(-34.919829498708,-1.83573964553602,326.315593435747));
#10161=CARTESIAN_POINT('Ctrl Pts',(-35.0709574919393,-1.83573964553603,
326.06166299344));
#10162=CARTESIAN_POINT('Ctrl Pts',(-35.2117363266656,-1.83573964553605,
325.800586363758));
#10163=CARTESIAN_POINT('Ctrl Pts',(-35.3429176445163,-1.83573964553607,
325.557308484605));
#10164=CARTESIAN_POINT('Ctrl Pts',(-35.4651065858305,-1.83573964553609,
325.307828880366));
#10165=CARTESIAN_POINT('Ctrl Pts',(-35.5734293953103,-1.8357396455361,325.054611439063));
#10166=CARTESIAN_POINT('Ctrl Pts',(-35.624205712254,-1.83573964553611,324.935915763452));
#10167=CARTESIAN_POINT('Ctrl Pts',(-35.6719358463144,-1.83573964553612,
324.816398306841));
#10168=CARTESIAN_POINT('Ctrl Pts',(-35.7161231976916,-1.83573964553612,
324.696308546926));
#10169=CARTESIAN_POINT('Ctrl Pts',(-35.7375264460149,-1.83573964553612,
324.638140069467));
#10170=CARTESIAN_POINT('Ctrl Pts',(-35.7580985605365,-1.83573964553612,
324.579837262752));
#10171=CARTESIAN_POINT('Ctrl Pts',(-35.7777835675407,-1.83573964553612,
324.521428110438));
#10172=CARTESIAN_POINT('Ctrl Pts',(-35.790121733712,-1.83573964553613,324.484818429424));
#10173=CARTESIAN_POINT('Ctrl Pts',(-35.8021114034735,-1.83573964553613,
324.448166965075));
#10174=CARTESIAN_POINT('Ctrl Pts',(-35.8137388658144,-1.83573964553613,
324.411480550089));
#10175=CARTESIAN_POINT('Ctrl Pts',(-35.8199545189524,-1.83573964553613,
324.391869217561));
#10176=CARTESIAN_POINT('Ctrl Pts',(-35.8260666681465,-1.83573964553613,
324.372247896694));
#10177=CARTESIAN_POINT('Ctrl Pts',(-35.832073225929,-1.83573964553613,324.352617625523));
#10178=CARTESIAN_POINT('Ctrl Pts',(-35.8354794513467,-1.83573964553613,
324.341485604316));
#10179=CARTESIAN_POINT('Ctrl Pts',(-35.8388527537894,-1.83573964553612,
324.330347382553));
#10180=CARTESIAN_POINT('Ctrl Pts',(-35.842195044056,-1.83573964553612,324.319195126364));
#10181=CARTESIAN_POINT('Ctrl Pts',(-35.904156576116,-1.83573964553612,324.112447410186));
#10182=CARTESIAN_POINT('Ctrl Pts',(-35.955206972034,-1.83573964553613,323.901705493671));
#10183=CARTESIAN_POINT('Ctrl Pts',(-35.991654591359,-1.83573964553613,323.688750751308));
#10184=CARTESIAN_POINT('Ctrl Pts',(-36.0214654326083,-1.83573964553613,
323.514573119533));
#10185=CARTESIAN_POINT('Ctrl Pts',(-36.0415060533855,-1.83573964553613,
323.33891554914));
#10186=CARTESIAN_POINT('Ctrl Pts',(-36.0497684509554,-1.83573964553613,
323.162717079327));
#10187=CARTESIAN_POINT('Ctrl Pts',(-36.0522529480809,-1.83573964553613,
323.109734323647));
#10188=CARTESIAN_POINT('Ctrl Pts',(-36.0536726122713,-1.83573964553613,
323.056702357695));
#10189=CARTESIAN_POINT('Ctrl Pts',(-36.0539733280531,-1.83573964553613,
323.003645833575));
#10190=CARTESIAN_POINT('Ctrl Pts',(-36.0541436617393,-1.83573964553613,
322.973593159648));
#10191=CARTESIAN_POINT('Ctrl Pts',(-36.0539549967846,-1.83573964553613,
322.943532598032));
#10192=CARTESIAN_POINT('Ctrl Pts',(-36.0533975407004,-1.83573964553613,
322.913468557433));
#10193=CARTESIAN_POINT('Ctrl Pts',(-36.0530871771216,-1.83573964553613,
322.896730408008));
#10194=CARTESIAN_POINT('Ctrl Pts',(-36.0526624997886,-1.83573964553613,
322.879991179246));
#10195=CARTESIAN_POINT('Ctrl Pts',(-36.0521218232439,-1.83573964553613,
322.863251624484));
#10196=CARTESIAN_POINT('Ctrl Pts',(-36.0517128308649,-1.83573964553613,
322.850589062382));
#10197=CARTESIAN_POINT('Ctrl Pts',(-36.0512373152779,-1.83573964553613,
322.83792418292));
#10198=CARTESIAN_POINT('Ctrl Pts',(-36.0506956710076,-1.83573964553613,
322.825279591146));
#10199=CARTESIAN_POINT('Ctrl Pts',(-36.0428318976773,-1.83573964553613,
322.641701163372));
#10200=CARTESIAN_POINT('Ctrl Pts',(-36.0210023687523,-1.83573964553613,
322.461375790017));
#10201=CARTESIAN_POINT('Ctrl Pts',(-35.984438433772,-1.83573964553612,322.284478185075));
#10202=CARTESIAN_POINT('Ctrl Pts',(-35.9498008213356,-1.83573964553611,
322.116900196432));
#10203=CARTESIAN_POINT('Ctrl Pts',(-35.9019401767507,-1.83573964553611,
321.952398681821));
#10204=CARTESIAN_POINT('Ctrl Pts',(-35.8402013746489,-1.83573964553611,
321.791073726073));
#10205=CARTESIAN_POINT('Ctrl Pts',(-35.8239901926768,-1.83573964553611,
321.74871352268));
#10206=CARTESIAN_POINT('Ctrl Pts',(-35.8068221660236,-1.83573964553611,
321.706572051959));
#10207=CARTESIAN_POINT('Ctrl Pts',(-35.7886854810261,-1.83573964553611,
321.664650526461));
#10208=CARTESIAN_POINT('Ctrl Pts',(-35.7836966569188,-1.83573964553611,
321.653119250649));
#10209=CARTESIAN_POINT('Ctrl Pts',(-35.7786345419672,-1.83573964553611,
321.641604614989));
#10210=CARTESIAN_POINT('Ctrl Pts',(-35.7734988909164,-1.83573964553611,
321.630106641422));
#10211=CARTESIAN_POINT('Ctrl Pts',(-35.7700958011473,-1.83573964553611,
321.622487619837));
#10212=CARTESIAN_POINT('Ctrl Pts',(-35.7666637923649,-1.83573964553611,
321.614883486877));
#10213=CARTESIAN_POINT('Ctrl Pts',(-35.7632047952331,-1.83573964553611,
321.60729809249));
#10214=CARTESIAN_POINT('Ctrl Pts',(-35.6868709731977,-1.83573964553611,
321.439902132573));
#10215=CARTESIAN_POINT('Ctrl Pts',(-35.5971163415451,-1.83573964553611,
321.281019102654));
#10216=CARTESIAN_POINT('Ctrl Pts',(-35.4959479809854,-1.83573964553611,
321.12997587918));
#10217=CARTESIAN_POINT('Ctrl Pts',(-35.4039568383216,-1.83573964553611,
320.992634138717));
#10218=CARTESIAN_POINT('Ctrl Pts',(-35.3025298409702,-1.83573964553611,
320.861773652812));
#10219=CARTESIAN_POINT('Ctrl Pts',(-35.1932091120446,-1.83573964553611,
320.736906185937));
#10220=CARTESIAN_POINT('Ctrl Pts',(-35.1419650203607,-1.83573964553611,
320.678374560839));
#10221=CARTESIAN_POINT('Ctrl Pts',(-35.0889868731899,-1.83573964553611,
320.621160091195));
#10222=CARTESIAN_POINT('Ctrl Pts',(-35.0344353428421,-1.83573964553611,
320.565214563772));
#10223=CARTESIAN_POINT('Ctrl Pts',(-35.0080119453299,-1.83573964553611,
320.538115948927));
#10224=CARTESIAN_POINT('Ctrl Pts',(-34.9812194168613,-1.83573964553611,
320.511315074697));
#10225=CARTESIAN_POINT('Ctrl Pts',(-34.9540760904638,-1.83573964553611,
320.484806595523));
#10226=CARTESIAN_POINT('Ctrl Pts',(-34.9452697370927,-1.83573964553611,
320.476206211343));
#10227=CARTESIAN_POINT('Ctrl Pts',(-34.9364264588272,-1.83573964553611,
320.467636605576));
#10228=CARTESIAN_POINT('Ctrl Pts',(-34.9275468826458,-1.83573964553611,
320.459097597761));
#10229=CARTESIAN_POINT('Ctrl Pts',(-34.9182349861886,-1.83573964553611,
320.450142850936));
#10230=CARTESIAN_POINT('Ctrl Pts',(-34.9088882279726,-1.83573964553611,
320.441226479291));
#10231=CARTESIAN_POINT('Ctrl Pts',(-34.8994801179544,-1.83573964553611,
320.432322702167));
#10232=CARTESIAN_POINT('Ctrl Pts',(-34.7581536133364,-1.83573964553611,
320.298572172423));
#10233=CARTESIAN_POINT('Ctrl Pts',(-34.6038513564271,-1.8357396455361,320.168510760348));
#10234=CARTESIAN_POINT('Ctrl Pts',(-34.4364491814111,-1.83573964553609,
320.041799621155));
#10235=CARTESIAN_POINT('Ctrl Pts',(-34.2593578809453,-1.83573964553607,
319.907754526335));
#10236=CARTESIAN_POINT('Ctrl Pts',(-34.0676058937315,-1.83573964553606,
319.777458308624));
#10237=CARTESIAN_POINT('Ctrl Pts',(-33.8609893372873,-1.83573964553604,
319.650529883203));
#10238=CARTESIAN_POINT('Ctrl Pts',(-33.635098772893,-1.83573964553603,319.511761073242));
#10239=CARTESIAN_POINT('Ctrl Pts',(-33.391439573106,-1.83573964553602,319.377016777585));
#10240=CARTESIAN_POINT('Ctrl Pts',(-33.1296933633902,-1.83573964553601,
319.245833289073));
#10241=CARTESIAN_POINT('Ctrl Pts',(-33.066169688179,-1.83573964553601,319.21399612388));
#10242=CARTESIAN_POINT('Ctrl Pts',(-33.0015805470171,-1.83573964553601,
319.182368871595));
#10243=CARTESIAN_POINT('Ctrl Pts',(-32.9359211723264,-1.83573964553601,
319.15094527135));
#10244=CARTESIAN_POINT('Ctrl Pts',(-32.927382150455,-1.83573964553601,319.146858622474));
#10245=CARTESIAN_POINT('Ctrl Pts',(-32.9188288323849,-1.83573964553601,
319.142777214983));
#10246=CARTESIAN_POINT('Ctrl Pts',(-32.9102355177821,-1.83573964553601,
319.138688853223));
#10247=CARTESIAN_POINT('Ctrl Pts',(-32.7983897862637,-1.83573964553601,
319.085477044647));
#10248=CARTESIAN_POINT('Ctrl Pts',(-32.6805626663053,-1.83573964553601,
319.031466453008));
#10249=CARTESIAN_POINT('Ctrl Pts',(-32.5560947943014,-1.83573964553601,
318.976659291702));
#10250=CARTESIAN_POINT('Ctrl Pts',(-32.4312856481312,-1.83573964553601,
318.921701856531));
#10251=CARTESIAN_POINT('Ctrl Pts',(-32.2997992729873,-1.83573964553601,
318.865943489233));
#10252=CARTESIAN_POINT('Ctrl Pts',(-32.1609188082923,-1.83573964553601,
318.809392801681));
#10253=CARTESIAN_POINT('Ctrl Pts',(-32.0194975723913,-1.83573964553601,
318.751807538397));
#10254=CARTESIAN_POINT('Ctrl Pts',(-31.8704092594458,-1.83573964553601,
318.693400697781));
#10255=CARTESIAN_POINT('Ctrl Pts',(-31.7128425891105,-1.83573964553601,
318.634187910249));
#10256=CARTESIAN_POINT('Ctrl Pts',(-31.5511994143238,-1.83573964553601,
318.573443192193));
#10257=CARTESIAN_POINT('Ctrl Pts',(-31.3806334401196,-1.83573964553601,
318.511850269096));
#10258=CARTESIAN_POINT('Ctrl Pts',(-31.200212177051,-1.83573964553601,318.44943297343));
#10259=CARTESIAN_POINT('Ctrl Pts',(-31.0112459120662,-1.83573964553601,
318.384059507842));
#10260=CARTESIAN_POINT('Ctrl Pts',(-30.8114685442404,-1.83573964553601,
318.317781667008));
#10261=CARTESIAN_POINT('Ctrl Pts',(-30.5997488998527,-1.83573964553601,
318.250635026041));
#10262=CARTESIAN_POINT('Ctrl Pts',(-30.3701849676304,-1.83573964553601,
318.177829089775));
#10263=CARTESIAN_POINT('Ctrl Pts',(-30.126580348697,-1.83573964553601,318.104001539579));
#10264=CARTESIAN_POINT('Ctrl Pts',(-29.867429065394,-1.83573964553601,318.029209289024));
#10265=CARTESIAN_POINT('Ctrl Pts',(-29.5544940093786,-1.83573964553601,
317.938894794655));
#10266=CARTESIAN_POINT('Ctrl Pts',(-29.2188882099064,-1.83573964553601,
317.847172910493));
#10267=CARTESIAN_POINT('Ctrl Pts',(-28.8578814451977,-1.83573964553601,
317.754167971317));
#10268=CARTESIAN_POINT('Ctrl Pts',(-28.5298192834568,-1.83573964553601,
317.669650437627));
#10269=CARTESIAN_POINT('Ctrl Pts',(-28.1807761284515,-1.83573964553601,
317.584073620011));
#10270=CARTESIAN_POINT('Ctrl Pts',(-27.8086957725647,-1.83573964553601,
317.497550185639));
#10271=CARTESIAN_POINT('Ctrl Pts',(-27.4831254611637,-1.83573964553601,
317.421842180563));
#10272=CARTESIAN_POINT('Ctrl Pts',(-27.1399151008274,-1.83573964553601,
317.345409648215));
#10273=CARTESIAN_POINT('Ctrl Pts',(-26.7777227702123,-1.83573964553602,
317.268340184405));
#10274=CARTESIAN_POINT('Ctrl Pts',(-26.4608044809241,-1.83573964553602,
317.200904403571));
#10275=CARTESIAN_POINT('Ctrl Pts',(-26.1293523138813,-1.83573964553602,
317.132981084406));
#10276=CARTESIAN_POINT('Ctrl Pts',(-25.7825143870751,-1.83573964553602,
317.064636847793));
#10277=CARTESIAN_POINT('Ctrl Pts',(-25.4790312011196,-1.83573964553602,
317.004835640756));
#10278=CARTESIAN_POINT('Ctrl Pts',(-25.1637682058098,-1.83573964553602,
316.944712240703));
#10279=CARTESIAN_POINT('Ctrl Pts',(-24.8361981433063,-1.83573964553602,
316.884316639796));
#10280=CARTESIAN_POINT('Ctrl Pts',(-24.530513916328,-1.83573964553602,316.82795623117));
#10281=CARTESIAN_POINT('Ctrl Pts',(-24.214111964592,-1.83573964553601,316.771358791136));
#10282=CARTESIAN_POINT('Ctrl Pts',(-23.8866071050454,-1.83573964553602,
316.714569487522));
#10283=CARTESIAN_POINT('Ctrl Pts',(-23.5723176576479,-1.83573964553602,
316.660071734799));
#10284=CARTESIAN_POINT('Ctrl Pts',(-23.2478029725362,-1.83573964553601,
316.605397287888));
#10285=CARTESIAN_POINT('Ctrl Pts',(-22.9127680347174,-1.83573964553602,
316.550590348815));
#10286=CARTESIAN_POINT('Ctrl Pts',(-22.5888443425662,-1.83573964553602,
316.497601051114));
#10287=CARTESIAN_POINT('Ctrl Pts',(-22.2550863795048,-1.83573964553602,
316.444487898802));
#10288=CARTESIAN_POINT('Ctrl Pts',(-21.9112747750118,-1.83573964553602,
316.39129498806));
#10289=CARTESIAN_POINT('Ctrl Pts',(-21.5769144833199,-1.83573964553602,
316.339564339883));
#10290=CARTESIAN_POINT('Ctrl Pts',(-21.2330455008927,-1.83573964553602,
316.287758252604));
#10291=CARTESIAN_POINT('Ctrl Pts',(-20.879514750595,-1.83573964553602,316.235921354704));
#10292=CARTESIAN_POINT('Ctrl Pts',(-20.5342625107455,-1.83573964553602,
316.185298303975));
#10293=CARTESIAN_POINT('Ctrl Pts',(-20.1797955310403,-1.83573964553602,
316.13464586032));
#10294=CARTESIAN_POINT('Ctrl Pts',(-19.8160210095592,-1.83573964553602,
316.084009629196));
#10295=CARTESIAN_POINT('Ctrl Pts',(-19.46163404477,-1.83573964553602,316.034680115454));
#10296=CARTESIAN_POINT('Ctrl Pts',(-19.098413653549,-1.83573964553602,315.985365984819));
#10297=CARTESIAN_POINT('Ctrl Pts',(-18.7263234961891,-1.83573964553602,
315.936113366434));
#10298=CARTESIAN_POINT('Ctrl Pts',(-18.3582593515104,-1.83573964553602,
315.887393661007));
#10299=CARTESIAN_POINT('Ctrl Pts',(-17.9815162269729,-1.83573964553602,
315.83873413412));
#10300=CARTESIAN_POINT('Ctrl Pts',(-17.596109528008,-1.83573964553602,315.790183476892));
#10301=CARTESIAN_POINT('Ctrl Pts',(-17.2136841826627,-1.83573964553602,
315.742008388325));
#10302=CARTESIAN_POINT('Ctrl Pts',(-16.8227287332923,-1.83573964553602,
315.693940487264));
#10303=CARTESIAN_POINT('Ctrl Pts',(-16.423309601714,-1.83573964553602,315.646031462909));
#10304=CARTESIAN_POINT('Ctrl Pts',(-16.2905773856919,-1.83573964553602,
315.630110665763));
#10305=CARTESIAN_POINT('Ctrl Pts',(-16.15691093349,-1.83573964553602,315.614207447801));
#10306=CARTESIAN_POINT('Ctrl Pts',(-16.022313954939,-1.83573964553602,315.598323807971));
#10307=CARTESIAN_POINT('',(-33.0349479481876,-1.83573964553602,325.551079813359));
#10308=CARTESIAN_POINT('',(-33.0293694032794,-1.83573964553602,325.547827590886));
#10309=CARTESIAN_POINT('Ctrl Pts',(-16.0223151822761,-1.83573964553602,
317.612324258224));
#10310=CARTESIAN_POINT('Ctrl Pts',(-16.1477973978183,-1.83573964553602,
317.627281546276));
#10311=CARTESIAN_POINT('Ctrl Pts',(-16.2739661013669,-1.83573964553602,
317.642433264547));
#10312=CARTESIAN_POINT('Ctrl Pts',(-16.4007776292659,-1.83573964553602,
317.65778048784));
#10313=CARTESIAN_POINT('Ctrl Pts',(-16.7384550918035,-1.83573964553602,
317.698647524965));
#10314=CARTESIAN_POINT('Ctrl Pts',(-17.0804884887966,-1.83573964553603,
317.740910768462));
#10315=CARTESIAN_POINT('Ctrl Pts',(-17.4258778156812,-1.83573964553603,
317.784588179341));
#10316=CARTESIAN_POINT('Ctrl Pts',(-17.7806192669341,-1.83573964553604,
317.829448245696));
#10317=CARTESIAN_POINT('Ctrl Pts',(-18.1389006976833,-1.83573964553604,
317.87580016583));
#10318=CARTESIAN_POINT('Ctrl Pts',(-18.4995828290648,-1.83573964553605,
317.923658900772));
#10319=CARTESIAN_POINT('Ctrl Pts',(-18.8743379902158,-1.83573964553605,
317.973384979125));
#10320=CARTESIAN_POINT('Ctrl Pts',(-19.2516846085092,-1.83573964553607,
318.024737842581));
#10321=CARTESIAN_POINT('Ctrl Pts',(-19.6302880901341,-1.83573964553608,
318.077728238319));
#10322=CARTESIAN_POINT('Ctrl Pts',(-20.0308257740179,-1.83573964553609,
318.133788605978));
#10323=CARTESIAN_POINT('Ctrl Pts',(-20.4327697742083,-1.8357396455361,318.19168188436));
#10324=CARTESIAN_POINT('Ctrl Pts',(-20.834482210606,-1.83573964553611,318.251412294469));
#10325=CARTESIAN_POINT('Ctrl Pts',(-21.303558974513,-1.83573964553612,318.321159070876));
#10326=CARTESIAN_POINT('Ctrl Pts',(-21.7723197118664,-1.83573964553613,
318.39341130996));
#10327=CARTESIAN_POINT('Ctrl Pts',(-22.23808360911,-1.83573964553615,318.468158799972));
#10328=CARTESIAN_POINT('Ctrl Pts',(-22.8064091100986,-1.83573964553616,
318.559365750447));
#10329=CARTESIAN_POINT('Ctrl Pts',(-23.3702689307725,-1.83573964553617,
318.654289363245));
#10330=CARTESIAN_POINT('Ctrl Pts',(-23.9247188275741,-1.83573964553618,
318.752869991931));
#10331=CARTESIAN_POINT('Ctrl Pts',(-24.3988170855096,-1.83573964553619,
318.837164180813));
#10332=CARTESIAN_POINT('Ctrl Pts',(-24.8660306052653,-1.8357396455362,318.924131605397));
#10333=CARTESIAN_POINT('Ctrl Pts',(-25.3232865256788,-1.8357396455362,319.013706084701));
#10334=CARTESIAN_POINT('Ctrl Pts',(-25.4090220107563,-1.8357396455362,319.030501299571));
#10335=CARTESIAN_POINT('Ctrl Pts',(-25.4944075808075,-1.8357396455362,319.047388089524));
#10336=CARTESIAN_POINT('Ctrl Pts',(-25.5794232403297,-1.8357396455362,319.064365907288));
#10337=CARTESIAN_POINT('Ctrl Pts',(-25.6227005251825,-1.8357396455362,319.073008478076));
#10338=CARTESIAN_POINT('Ctrl Pts',(-25.6658819558488,-1.8357396455362,319.081674636569));
#10339=CARTESIAN_POINT('Ctrl Pts',(-25.7089649060401,-1.8357396455362,319.090364306988));
#10340=CARTESIAN_POINT('Ctrl Pts',(-25.7317114794517,-1.8357396455362,319.094952206034));
#10341=CARTESIAN_POINT('Ctrl Pts',(-25.7544306011717,-1.8357396455362,319.099546659082));
#10342=CARTESIAN_POINT('Ctrl Pts',(-25.7771218856057,-1.8357396455362,319.104147654706));
#10343=CARTESIAN_POINT('Ctrl Pts',(-25.798394351303,-1.8357396455362,319.108460963715));
#10344=CARTESIAN_POINT('Ctrl Pts',(-25.8196336740054,-1.8357396455362,319.112778264217));
#10345=CARTESIAN_POINT('Ctrl Pts',(-25.8408363513149,-1.8357396455362,319.117098867872));
#10346=CARTESIAN_POINT('Ctrl Pts',(-26.117190526685,-1.8357396455362,319.173413306037));
#10347=CARTESIAN_POINT('Ctrl Pts',(-26.3875181930021,-1.8357396455362,319.230327749865));
#10348=CARTESIAN_POINT('Ctrl Pts',(-26.6518879881453,-1.8357396455362,319.287913666536));
#10349=CARTESIAN_POINT('Ctrl Pts',(-26.9038922118028,-1.8357396455362,319.342806072897));
#10350=CARTESIAN_POINT('Ctrl Pts',(-27.1504829743502,-1.8357396455362,319.398308654903));
#10351=CARTESIAN_POINT('Ctrl Pts',(-27.3916728179156,-1.8357396455362,319.454489746202));
#10352=CARTESIAN_POINT('Ctrl Pts',(-27.6271052020578,-1.8357396455362,319.509329734788));
#10353=CARTESIAN_POINT('Ctrl Pts',(-27.8573916738498,-1.8357396455362,319.564816243724));
#10354=CARTESIAN_POINT('Ctrl Pts',(-28.0824954546864,-1.8357396455362,319.621018670888));
#10355=CARTESIAN_POINT('Ctrl Pts',(-28.3002562087911,-1.8357396455362,319.675387739575));
#10356=CARTESIAN_POINT('Ctrl Pts',(-28.5131670000565,-1.8357396455362,319.730426803238));
#10357=CARTESIAN_POINT('Ctrl Pts',(-28.7211462451106,-1.8357396455362,319.786203917586));
#10358=CARTESIAN_POINT('Ctrl Pts',(-28.8297860424903,-1.8357396455362,319.815339586386));
#10359=CARTESIAN_POINT('Ctrl Pts',(-28.9370794045402,-1.8357396455362,319.844676724422));
#10360=CARTESIAN_POINT('Ctrl Pts',(-29.043009016516,-1.8357396455362,319.874225600227));
#10361=CARTESIAN_POINT('Ctrl Pts',(-29.2397507640582,-1.8357396455362,319.92910635883));
#10362=CARTESIAN_POINT('Ctrl Pts',(-29.4316765956865,-1.8357396455362,319.98486773198));
#10363=CARTESIAN_POINT('Ctrl Pts',(-29.6187127167007,-1.8357396455362,320.041439421539));
#10364=CARTESIAN_POINT('Ctrl Pts',(-29.8024953509048,-1.8357396455362,320.097027048528));
#10365=CARTESIAN_POINT('Ctrl Pts',(-29.9815570165904,-1.8357396455362,320.153397216642));
#10366=CARTESIAN_POINT('Ctrl Pts',(-30.1557786611949,-1.8357396455362,320.210481790954));
#10367=CARTESIAN_POINT('Ctrl Pts',(-30.3269354514096,-1.8357396455362,320.266562150729));
#10368=CARTESIAN_POINT('Ctrl Pts',(-30.4934211174452,-1.8357396455362,320.323332157974));
#10369=CARTESIAN_POINT('Ctrl Pts',(-30.6550734539028,-1.8357396455362,320.380723420614));
#10370=CARTESIAN_POINT('Ctrl Pts',(-30.813866991154,-1.8357396455362,320.437099726714));
#10371=CARTESIAN_POINT('Ctrl Pts',(-30.9679967454257,-1.8357396455362,320.49407565197));
#10372=CARTESIAN_POINT('Ctrl Pts',(-31.1172593976607,-1.8357396455362,320.551580492726));
#10373=CARTESIAN_POINT('Ctrl Pts',(-31.2638800782195,-1.8357396455362,320.608067489043));
#10374=CARTESIAN_POINT('Ctrl Pts',(-31.4058045324441,-1.8357396455362,320.665064975756));
#10375=CARTESIAN_POINT('Ctrl Pts',(-31.542790261857,-1.8357396455362,320.722498194282));
#10376=CARTESIAN_POINT('Ctrl Pts',(-31.5984863479931,-1.8357396455362,320.745849571829));
#10377=CARTESIAN_POINT('Ctrl Pts',(-31.6533654258363,-1.8357396455362,320.769272878874));
#10378=CARTESIAN_POINT('Ctrl Pts',(-31.7074087147834,-1.8357396455362,320.792762636528));
#10379=CARTESIAN_POINT('Ctrl Pts',(-31.7310526536978,-1.8357396455362,320.803039405501));
#10380=CARTESIAN_POINT('Ctrl Pts',(-31.7545365983725,-1.8357396455362,320.813328889837));
#10381=CARTESIAN_POINT('Ctrl Pts',(-31.7778588863295,-1.8357396455362,320.823630612852));
#10382=CARTESIAN_POINT('Ctrl Pts',(-31.7887912088093,-1.8357396455362,320.828459545515));
#10383=CARTESIAN_POINT('Ctrl Pts',(-31.7996880102247,-1.8357396455362,320.833291167181));
#10384=CARTESIAN_POINT('Ctrl Pts',(-31.8105491151427,-1.8357396455362,320.838125427887));
#10385=CARTESIAN_POINT('Ctrl Pts',(-31.8186120876275,-1.8357396455362,320.84171424425));
#10386=CARTESIAN_POINT('Ctrl Pts',(-31.8266553871769,-1.8357396455362,320.845304515018));
#10387=CARTESIAN_POINT('Ctrl Pts',(-31.834678941052,-1.8357396455362,320.848896219547));
#10388=CARTESIAN_POINT('Ctrl Pts',(-31.8383935430248,-1.8357396455362,320.850559042897));
#10389=CARTESIAN_POINT('Ctrl Pts',(-31.8421110078627,-1.8357396455362,320.852225347479));
#10390=CARTESIAN_POINT('Ctrl Pts',(-31.8458365934522,-1.8357396455362,320.853897526144));
#10391=CARTESIAN_POINT('Ctrl Pts',(-31.8943141308875,-1.8357396455362,320.875656012666));
#10392=CARTESIAN_POINT('Ctrl Pts',(-31.9438878817209,-1.8357396455362,320.898282844771));
#10393=CARTESIAN_POINT('Ctrl Pts',(-31.9945004898157,-1.8357396455362,320.921848711034));
#10394=CARTESIAN_POINT('Ctrl Pts',(-32.0435915780867,-1.83573964553619,
320.944706138548));
#10395=CARTESIAN_POINT('Ctrl Pts',(-32.0936601971404,-1.8357396455362,320.968447061434));
#10396=CARTESIAN_POINT('Ctrl Pts',(-32.1446063538921,-1.8357396455362,320.993131362249));
#10397=CARTESIAN_POINT('Ctrl Pts',(-32.1940839096517,-1.83573964553619,
321.01710410029));
#10398=CARTESIAN_POINT('Ctrl Pts',(-32.244389327626,-1.83573964553619,321.04196668715));
#10399=CARTESIAN_POINT('Ctrl Pts',(-32.2953825917274,-1.83573964553619,
321.06776848529));
#10400=CARTESIAN_POINT('Ctrl Pts',(-32.3464999294076,-1.83573964553619,
321.09363306273));
#10401=CARTESIAN_POINT('Ctrl Pts',(-32.3983089480635,-1.83573964553619,
321.120441552904));
#10402=CARTESIAN_POINT('Ctrl Pts',(-32.4506138713051,-1.83573964553619,
321.148236549717));
#10403=CARTESIAN_POINT('Ctrl Pts',(-32.4993675440086,-1.83573964553618,
321.17414440109));
#10404=CARTESIAN_POINT('Ctrl Pts',(-32.5485518829854,-1.83573964553618,
321.20090937913));
#10405=CARTESIAN_POINT('Ctrl Pts',(-32.5979598565244,-1.83573964553618,
321.228558830698));
#10406=CARTESIAN_POINT('Ctrl Pts',(-32.6463013406213,-1.83573964553618,
321.255611458594));
#10407=CARTESIAN_POINT('Ctrl Pts',(-32.6948571014369,-1.83573964553618,
321.283510876491));
#10408=CARTESIAN_POINT('Ctrl Pts',(-32.7433845017131,-1.83573964553617,
321.312274677328));
#10409=CARTESIAN_POINT('Ctrl Pts',(-32.7904668306801,-1.83573964553617,
321.340181936437));
#10410=CARTESIAN_POINT('Ctrl Pts',(-32.8375225714865,-1.83573964553617,
321.368902940896));
#10411=CARTESIAN_POINT('Ctrl Pts',(-32.8842816827013,-1.83573964553617,
321.39844495528));
#10412=CARTESIAN_POINT('Ctrl Pts',(-32.8986071664417,-1.83573964553617,
321.407495675787));
#10413=CARTESIAN_POINT('Ctrl Pts',(-32.9129044496341,-1.83573964553617,
321.416623388818));
#10414=CARTESIAN_POINT('Ctrl Pts',(-32.9271647914283,-1.83573964553617,
321.425828112808));
#10415=CARTESIAN_POINT('Ctrl Pts',(-32.9894393416746,-1.83573964553616,
321.466024908572));
#10416=CARTESIAN_POINT('Ctrl Pts',(-33.0508307284169,-1.83573964553616,
321.507320268099));
#10417=CARTESIAN_POINT('Ctrl Pts',(-33.1107858604198,-1.83573964553616,
321.549628247802));
#10418=CARTESIAN_POINT('Ctrl Pts',(-33.1720746579612,-1.83573964553616,
321.592877342846));
#10419=CARTESIAN_POINT('Ctrl Pts',(-33.2318608770518,-1.83573964553616,
321.63718525381));
#10420=CARTESIAN_POINT('Ctrl Pts',(-33.2895248559089,-1.83573964553616,
321.68241432941));
#10421=CARTESIAN_POINT('Ctrl Pts',(-33.3193726179928,-1.83573964553616,
321.705825594371));
#10422=CARTESIAN_POINT('Ctrl Pts',(-33.3486514607266,-1.83573964553616,
321.729482861706));
#10423=CARTESIAN_POINT('Ctrl Pts',(-33.3772752459844,-1.83573964553616,
321.753361462868));
#10424=CARTESIAN_POINT('Ctrl Pts',(-33.3842931760298,-1.83573964553616,
321.759215976903));
#10425=CARTESIAN_POINT('Ctrl Pts',(-33.391271734033,-1.83573964553616,321.765083776658));
#10426=CARTESIAN_POINT('Ctrl Pts',(-33.3982096632514,-1.83573964553616,
321.77096446054));
#10427=CARTESIAN_POINT('Ctrl Pts',(-33.402477062095,-1.83573964553616,321.774581566281));
#10428=CARTESIAN_POINT('Ctrl Pts',(-33.4067290901233,-1.83573964553616,
321.778203546127));
#10429=CARTESIAN_POINT('Ctrl Pts',(-33.4109654563272,-1.83573964553616,
321.781830303713));
#10430=CARTESIAN_POINT('Ctrl Pts',(-33.4148431507004,-1.83573964553616,
321.785150001966));
#10431=CARTESIAN_POINT('Ctrl Pts',(-33.4187026046589,-1.83573964553616,
321.788469247158));
#10432=CARTESIAN_POINT('Ctrl Pts',(-33.4225714468093,-1.83573964553616,
321.791812128747));
#10433=CARTESIAN_POINT('Ctrl Pts',(-33.4452246673039,-1.83573964553616,
321.811385693854));
#10434=CARTESIAN_POINT('Ctrl Pts',(-33.4680629603235,-1.83573964553616,
321.831651975973));
#10435=CARTESIAN_POINT('Ctrl Pts',(-33.4910161306369,-1.83573964553615,
321.852677020657));
#10436=CARTESIAN_POINT('Ctrl Pts',(-33.5136942685448,-1.83573964553615,
321.87345013637));
#10437=CARTESIAN_POINT('Ctrl Pts',(-33.536484452749,-1.83573964553614,321.894964144132));
#10438=CARTESIAN_POINT('Ctrl Pts',(-33.5592711467275,-1.83573964553614,
321.917262733865));
#10439=CARTESIAN_POINT('Ctrl Pts',(-33.5821431274893,-1.83573964553613,
321.939644783488));
#10440=CARTESIAN_POINT('Ctrl Pts',(-33.6050114507462,-1.83573964553612,
321.962817602908));
#10441=CARTESIAN_POINT('Ctrl Pts',(-33.6277123054661,-1.83573964553611,
321.98680122055));
#10442=CARTESIAN_POINT('Ctrl Pts',(-33.6506692348741,-1.8357396455361,322.011055382957));
#10443=CARTESIAN_POINT('Ctrl Pts',(-33.6734545419924,-1.8357396455361,322.03613915095));
#10444=CARTESIAN_POINT('Ctrl Pts',(-33.6958544071543,-1.83573964553609,
322.062043130631));
#10445=CARTESIAN_POINT('Ctrl Pts',(-33.7187953743038,-1.83573964553608,
322.088572859386));
#10446=CARTESIAN_POINT('Ctrl Pts',(-33.7413313269736,-1.83573964553607,
322.11596352265));
#10447=CARTESIAN_POINT('Ctrl Pts',(-33.7631941644085,-1.83573964553606,
322.144165673376));
#10448=CARTESIAN_POINT('Ctrl Pts',(-33.7848498866783,-1.83573964553606,
322.172100654155));
#10449=CARTESIAN_POINT('Ctrl Pts',(-33.8058437524814,-1.83573964553605,
322.200832290472));
#10450=CARTESIAN_POINT('Ctrl Pts',(-33.8258944208442,-1.83573964553605,
322.230266536138));
#10451=CARTESIAN_POINT('Ctrl Pts',(-33.8453345267723,-1.83573964553604,
322.258804480276));
#10452=CARTESIAN_POINT('Ctrl Pts',(-33.8638861983463,-1.83573964553604,
322.288003201187));
#10453=CARTESIAN_POINT('Ctrl Pts',(-33.8812971531608,-1.83573964553604,
322.317728145159));
#10454=CARTESIAN_POINT('Ctrl Pts',(-33.8842353512208,-1.83573964553604,
322.322744399215));
#10455=CARTESIAN_POINT('Ctrl Pts',(-33.8871411114321,-1.83573964553604,
322.327775517039));
#10456=CARTESIAN_POINT('Ctrl Pts',(-33.8900132952667,-1.83573964553604,
322.332820698899));
#10457=CARTESIAN_POINT('Ctrl Pts',(-33.8922620434555,-1.83573964553604,
322.336770774598));
#10458=CARTESIAN_POINT('Ctrl Pts',(-33.8944852638419,-1.83573964553604,
322.340720790062));
#10459=CARTESIAN_POINT('Ctrl Pts',(-33.8966822147502,-1.83573964553604,
322.344669336975));
#10460=CARTESIAN_POINT('Ctrl Pts',(-33.908306979514,-1.83573964553604,322.365562352312));
#10461=CARTESIAN_POINT('Ctrl Pts',(-33.9191931896151,-1.83573964553604,
322.386415387575));
#10462=CARTESIAN_POINT('Ctrl Pts',(-33.9292861005445,-1.83573964553604,
322.407067430352));
#10463=CARTESIAN_POINT('Ctrl Pts',(-33.9417031850838,-1.83573964553604,
322.432475180689));
#10464=CARTESIAN_POINT('Ctrl Pts',(-33.9535747838004,-1.83573964553603,
322.458172095153));
#10465=CARTESIAN_POINT('Ctrl Pts',(-33.9646867938464,-1.83573964553603,
322.48422003015));
#10466=CARTESIAN_POINT('Ctrl Pts',(-33.9758929094462,-1.83573964553603,
322.510488560281));
#10467=CARTESIAN_POINT('Ctrl Pts',(-33.9863256532958,-1.83573964553603,
322.537116716453));
#10468=CARTESIAN_POINT('Ctrl Pts',(-33.9958101702624,-1.83573964553603,
322.564189811733));
#10469=CARTESIAN_POINT('Ctrl Pts',(-34.0044657106833,-1.83573964553603,
322.588896633529));
#10470=CARTESIAN_POINT('Ctrl Pts',(-34.0123316649783,-1.83573964553602,
322.613975863777));
#10471=CARTESIAN_POINT('Ctrl Pts',(-34.0193159260718,-1.83573964553602,
322.639478830175));
#10472=CARTESIAN_POINT('Ctrl Pts',(-34.0257653553784,-1.83573964553602,
322.663028863126));
#10473=CARTESIAN_POINT('Ctrl Pts',(-34.0314631555427,-1.83573964553602,
322.686941105851));
#10474=CARTESIAN_POINT('Ctrl Pts',(-34.0363709590321,-1.83573964553602,
322.711226053297));
#10475=CARTESIAN_POINT('Ctrl Pts',(-34.041025494538,-1.83573964553602,322.734257772149));
#10476=CARTESIAN_POINT('Ctrl Pts',(-34.0449696036042,-1.83573964553602,
322.757625216962));
#10477=CARTESIAN_POINT('Ctrl Pts',(-34.0482003522234,-1.83573964553602,
322.781299822668));
#10478=CARTESIAN_POINT('Ctrl Pts',(-34.0501436708371,-1.83573964553602,
322.795540268882));
#10479=CARTESIAN_POINT('Ctrl Pts',(-34.0518290402368,-1.83573964553602,
322.809886093616));
#10480=CARTESIAN_POINT('Ctrl Pts',(-34.0532629695465,-1.83573964553602,
322.824344280636));
#10481=CARTESIAN_POINT('Ctrl Pts',(-34.0565952221417,-1.83573964553602,
322.857943099554));
#10482=CARTESIAN_POINT('Ctrl Pts',(-34.0585719809737,-1.83573964553602,
322.892167056002));
#10483=CARTESIAN_POINT('Ctrl Pts',(-34.0592900193062,-1.83573964553602,
322.927181258509));
#10484=CARTESIAN_POINT('Ctrl Pts',(-34.0600957471952,-1.83573964553602,
322.966471527839));
#10485=CARTESIAN_POINT('Ctrl Pts',(-34.0593169296225,-1.83573964553602,
323.006756557858));
#10486=CARTESIAN_POINT('Ctrl Pts',(-34.0570826346808,-1.83573964553602,
323.04820125649));
#10487=CARTESIAN_POINT('Ctrl Pts',(-34.0546549635249,-1.83573964553602,
323.093232956449));
#10488=CARTESIAN_POINT('Ctrl Pts',(-34.0505094908001,-1.83573964553602,
323.139632603362));
#10489=CARTESIAN_POINT('Ctrl Pts',(-34.0447957566754,-1.83573964553602,
323.187547675021));
#10490=CARTESIAN_POINT('Ctrl Pts',(-34.038259975017,-1.83573964553602,323.242356393747));
#10491=CARTESIAN_POINT('Ctrl Pts',(-34.0296733436094,-1.83573964553602,
323.299146247536));
#10492=CARTESIAN_POINT('Ctrl Pts',(-34.0192255510742,-1.83573964553602,
323.358080505269));
#10493=CARTESIAN_POINT('Ctrl Pts',(-34.0170778601807,-1.83573964553602,
323.370195271926));
#10494=CARTESIAN_POINT('Ctrl Pts',(-34.0148513871182,-1.83573964553602,
323.382400539659));
#10495=CARTESIAN_POINT('Ctrl Pts',(-34.0125475629435,-1.83573964553602,
323.394697592393));
#10496=CARTESIAN_POINT('Ctrl Pts',(-34.0041018612148,-1.83573964553602,
323.439777959496));
#10497=CARTESIAN_POINT('Ctrl Pts',(-33.9942378325614,-1.83573964553602,
323.485814537124));
#10498=CARTESIAN_POINT('Ctrl Pts',(-33.9830516029654,-1.83573964553602,
323.532667514042));
#10499=CARTESIAN_POINT('Ctrl Pts',(-33.9774997327527,-1.83573964553602,
323.555921251567));
#10500=CARTESIAN_POINT('Ctrl Pts',(-33.9716218371869,-1.83573964553602,
323.579376834424));
#10501=CARTESIAN_POINT('Ctrl Pts',(-33.9654276732709,-1.83573964553602,
323.603021343023));
#10502=CARTESIAN_POINT('Ctrl Pts',(-33.9632700493645,-1.83573964553602,
323.611257475889));
#10503=CARTESIAN_POINT('Ctrl Pts',(-33.9610740391173,-1.83573964553602,
323.619516555429));
#10504=CARTESIAN_POINT('Ctrl Pts',(-33.9588400165219,-1.83573964553602,
323.627798109298));
#10505=CARTESIAN_POINT('Ctrl Pts',(-33.9564896033297,-1.83573964553602,
323.636511124783));
#10506=CARTESIAN_POINT('Ctrl Pts',(-33.9540990870536,-1.83573964553602,
323.645241639339));
#10507=CARTESIAN_POINT('Ctrl Pts',(-33.9516709686306,-1.83573964553602,
323.65398245155));
#10508=CARTESIAN_POINT('Ctrl Pts',(-33.9357853389242,-1.83573964553602,
323.711168009224));
#10509=CARTESIAN_POINT('Ctrl Pts',(-33.9182697075581,-1.83573964553602,
323.768868124603));
#10510=CARTESIAN_POINT('Ctrl Pts',(-33.8993853314942,-1.83573964553602,
323.826715308049));
#10511=CARTESIAN_POINT('Ctrl Pts',(-33.8800632346799,-1.83573964553602,
323.885903330742));
#10512=CARTESIAN_POINT('Ctrl Pts',(-33.8593084218265,-1.83573964553602,
323.945245508614));
#10513=CARTESIAN_POINT('Ctrl Pts',(-33.8373921670454,-1.83573964553602,
324.004402817836));
#10514=CARTESIAN_POINT('Ctrl Pts',(-33.8149747048381,-1.83573964553602,
324.064913007967));
#10515=CARTESIAN_POINT('Ctrl Pts',(-33.7913422861375,-1.83573964553602,
324.125229980845));
#10516=CARTESIAN_POINT('Ctrl Pts',(-33.7667730232481,-1.83573964553602,
324.185044365047));
#10517=CARTESIAN_POINT('Ctrl Pts',(-33.7416528239998,-1.83573964553602,
324.246200015334));
#10518=CARTESIAN_POINT('Ctrl Pts',(-33.7155535047727,-1.83573964553602,
324.306830500987));
#10519=CARTESIAN_POINT('Ctrl Pts',(-33.688756410067,-1.83573964553602,324.366657164168));
#10520=CARTESIAN_POINT('Ctrl Pts',(-33.6610730441396,-1.83573964553602,
324.428462498934));
#10521=CARTESIAN_POINT('Ctrl Pts',(-33.6326452286528,-1.83573964553602,
324.489410106731));
#10522=CARTESIAN_POINT('Ctrl Pts',(-33.6037627924071,-1.83573964553602,
324.549244951856));
#10523=CARTESIAN_POINT('Ctrl Pts',(-33.5743135645162,-1.83573964553602,
324.610254001608));
#10524=CARTESIAN_POINT('Ctrl Pts',(-33.5443918862764,-1.83573964553602,
324.670106451295));
#10525=CARTESIAN_POINT('Ctrl Pts',(-33.5142808658538,-1.83573964553602,
324.728582005185));
#10526=CARTESIAN_POINT('Ctrl Pts',(-33.4835938597027,-1.83573964553602,
324.788176122446));
#10527=CARTESIAN_POINT('Ctrl Pts',(-33.4527103648113,-1.83573964553602,
324.846340431949));
#10528=CARTESIAN_POINT('Ctrl Pts',(-33.4219025092202,-1.83573964553602,
324.902889128396));
#10529=CARTESIAN_POINT('Ctrl Pts',(-33.3905174326719,-1.83573964553602,
324.960497330351));
#10530=CARTESIAN_POINT('Ctrl Pts',(-33.3592109971336,-1.83573964553602,
325.016429079736));
#10531=CARTESIAN_POINT('Ctrl Pts',(-33.3282402415969,-1.83573964553602,
325.070532506465));
#10532=CARTESIAN_POINT('Ctrl Pts',(-33.2964229457686,-1.83573964553602,
325.12611477121));
#10533=CARTESIAN_POINT('Ctrl Pts',(-33.2649600954318,-1.83573964553602,
325.179767610976));
#10534=CARTESIAN_POINT('Ctrl Pts',(-33.2340958895624,-1.83573964553602,
325.2313693393));
#10535=CARTESIAN_POINT('Ctrl Pts',(-33.2027399820095,-1.83573964553602,
325.28379314148));
#10536=CARTESIAN_POINT('Ctrl Pts',(-33.1720020130319,-1.83573964553602,
325.334100243464));
#10537=CARTESIAN_POINT('Ctrl Pts',(-33.1421012133259,-1.83573964553602,
325.382202871795));
#10538=CARTESIAN_POINT('Ctrl Pts',(-33.1115143190432,-1.83573964553602,
325.431409248278));
#10539=CARTESIAN_POINT('Ctrl Pts',(-33.0818035308545,-1.83573964553602,
325.478309060226));
#10540=CARTESIAN_POINT('Ctrl Pts',(-33.0531641026355,-1.83573964553602,
325.522845750499));
#10541=CARTESIAN_POINT('Ctrl Pts',(-33.0470426896219,-1.83573964553602,
325.532365056308));
#10542=CARTESIAN_POINT('Ctrl Pts',(-33.0409700794532,-1.83573964553602,
325.541776528307));
#10543=CARTESIAN_POINT('Ctrl Pts',(-33.0349479481876,-1.83573964553602,
325.551079813359));
#10544=CARTESIAN_POINT('Ctrl Pts',(16.317900533139,-13.,313.50573217442));
#10545=CARTESIAN_POINT('Ctrl Pts',(16.317900533139,9.8,313.50573217442));
#10546=CARTESIAN_POINT('Ctrl Pts',(15.6278893738391,-13.,313.517231811529));
#10547=CARTESIAN_POINT('Ctrl Pts',(15.6278893738391,9.8,313.517231811529));
#10548=CARTESIAN_POINT('Ctrl Pts',(14.2382065932492,-13.,313.544340068234));
#10549=CARTESIAN_POINT('Ctrl Pts',(14.2382065932492,9.8,313.544340068234));
#10550=CARTESIAN_POINT('Ctrl Pts',(12.1247011523636,-13.,313.597329370257));
#10551=CARTESIAN_POINT('Ctrl Pts',(12.1247011523636,9.8,313.597329370257));
#10552=CARTESIAN_POINT('Ctrl Pts',(9.24849377203438,-13.,313.692736456781));
#10553=CARTESIAN_POINT('Ctrl Pts',(9.24849377203438,9.8,313.692736456781));
#10554=CARTESIAN_POINT('Ctrl Pts',(5.55693877490966,-13.,313.853990642));
#10555=CARTESIAN_POINT('Ctrl Pts',(5.55693877490966,9.8,313.853990642));
#10556=CARTESIAN_POINT('Ctrl Pts',(1.77365151465576,-13.,314.058420030254));
#10557=CARTESIAN_POINT('Ctrl Pts',(1.77365151465576,9.8,314.058420030254));
#10558=CARTESIAN_POINT('Ctrl Pts',(-2.09023353797942,-13.,314.307572958727));
#10559=CARTESIAN_POINT('Ctrl Pts',(-2.09023353797942,9.8,314.307572958727));
#10560=CARTESIAN_POINT('Ctrl Pts',(-6.01421082656319,-13.,314.603269922693));
#10561=CARTESIAN_POINT('Ctrl Pts',(-6.01421082656319,9.8,314.603269922693));
#10562=CARTESIAN_POINT('Ctrl Pts',(-9.96528300844179,-13.,314.947459907816));
#10563=CARTESIAN_POINT('Ctrl Pts',(-9.96528300844179,9.8,314.947459907816));
#10564=CARTESIAN_POINT('Ctrl Pts',(-13.8949806972268,-13.,315.342078621379));
#10565=CARTESIAN_POINT('Ctrl Pts',(-13.8949806972268,9.8,315.342078621379));
#10566=CARTESIAN_POINT('Ctrl Pts',(-17.7352861120235,-13.,315.788771798629));
#10567=CARTESIAN_POINT('Ctrl Pts',(-17.7352861120235,9.8,315.788771798629));
#10568=CARTESIAN_POINT('Ctrl Pts',(-21.4049153651519,-13.,316.289764409719));
#10569=CARTESIAN_POINT('Ctrl Pts',(-21.4049153651519,9.8,316.289764409719));
#10570=CARTESIAN_POINT('Ctrl Pts',(-24.816789975018,-13.,316.848860723812));
#10571=CARTESIAN_POINT('Ctrl Pts',(-24.816789975018,9.8,316.848860723812));
#10572=CARTESIAN_POINT('Ctrl Pts',(-27.8849099804094,-13.,317.472300272892));
#10573=CARTESIAN_POINT('Ctrl Pts',(-27.8849099804094,9.8,317.472300272892));
#10574=CARTESIAN_POINT('Ctrl Pts',(-30.5321818074848,-13.,318.169788020995));
#10575=CARTESIAN_POINT('Ctrl Pts',(-30.5321818074848,9.8,318.169788020995));
#10576=CARTESIAN_POINT('Ctrl Pts',(-32.6972316847666,-13.,318.955110299069));
#10577=CARTESIAN_POINT('Ctrl Pts',(-32.6972316847666,9.8,318.955110299069));
#10578=CARTESIAN_POINT('Ctrl Pts',(-34.3449909415671,-13.,319.847716424401));
#10579=CARTESIAN_POINT('Ctrl Pts',(-34.3449909415671,9.8,319.847716424401));
#10580=CARTESIAN_POINT('Ctrl Pts',(-35.4659463455679,-13.,320.870731328741));
#10581=CARTESIAN_POINT('Ctrl Pts',(-35.4659463455679,9.8,320.870731328741));
#10582=CARTESIAN_POINT('Ctrl Pts',(-36.0649390676042,-13.,322.045906266434));
#10583=CARTESIAN_POINT('Ctrl Pts',(-36.0649390676042,9.8,322.045906266434));
#10584=CARTESIAN_POINT('Ctrl Pts',(-36.1525158245396,-13.,323.376843256979));
#10585=CARTESIAN_POINT('Ctrl Pts',(-36.1525158245396,9.8,323.376843256979));
#10586=CARTESIAN_POINT('Ctrl Pts',(-35.8309106944867,-13.,324.574753662996));
#10587=CARTESIAN_POINT('Ctrl Pts',(-35.8309106944867,9.8,324.574753662996));
#10588=CARTESIAN_POINT('Ctrl Pts',(-35.3753093664648,-13.,325.545731390974));
#10589=CARTESIAN_POINT('Ctrl Pts',(-35.3753093664648,9.8,325.545731390974));
#10590=CARTESIAN_POINT('Ctrl Pts',(-34.9799772611192,-13.,326.221291010618));
#10591=CARTESIAN_POINT('Ctrl Pts',(-34.9799772611192,9.8,326.221291010618));
#10592=CARTESIAN_POINT('Ctrl Pts',(-34.764378631884,-13.,326.559316446249));
#10593=CARTESIAN_POINT('Ctrl Pts',(-34.764378631884,9.8,326.559316446249));
#10594=CARTESIAN_POINT('',(-34.7643786318829,6.,326.55931644625));
#10595=CARTESIAN_POINT('',(-34.7643786318829,-13.,326.55931644625));
#10596=CARTESIAN_POINT('',(-20.0405545273386,6.,316.115431789383));
#10597=CARTESIAN_POINT('Ctrl Pts',(-20.0405545273386,6.,316.115431789383));
#10598=CARTESIAN_POINT('Ctrl Pts',(-20.3036630893018,6.,316.152450462513));
#10599=CARTESIAN_POINT('Ctrl Pts',(-21.2854516430835,6.,316.292780715073));
#10600=CARTESIAN_POINT('Ctrl Pts',(-22.949299720497,6.,316.545285451221));
#10601=CARTESIAN_POINT('Ctrl Pts',(-25.2075030604738,6.,316.92825331256));
#10602=CARTESIAN_POINT('Ctrl Pts',(-27.8849099804094,6.,317.472300272892));
#10603=CARTESIAN_POINT('Ctrl Pts',(-30.5321818074848,6.,318.169788020995));
#10604=CARTESIAN_POINT('Ctrl Pts',(-32.6972316847666,6.,318.955110299069));
#10605=CARTESIAN_POINT('Ctrl Pts',(-34.3449909415671,6.,319.847716424401));
#10606=CARTESIAN_POINT('Ctrl Pts',(-35.4659463455679,6.,320.870731328741));
#10607=CARTESIAN_POINT('Ctrl Pts',(-36.0649390676042,6.,322.045906266434));
#10608=CARTESIAN_POINT('Ctrl Pts',(-36.1525158245396,6.,323.376843256979));
#10609=CARTESIAN_POINT('Ctrl Pts',(-35.8309106944867,6.,324.574753662996));
#10610=CARTESIAN_POINT('Ctrl Pts',(-35.3753093664648,6.,325.545731390973));
#10611=CARTESIAN_POINT('Ctrl Pts',(-34.9799772611192,6.,326.221291010618));
#10612=CARTESIAN_POINT('Ctrl Pts',(-34.764378631884,6.,326.559316446249));
#10613=CARTESIAN_POINT('',(16.317900533139,6.,313.50573217442));
#10614=CARTESIAN_POINT('Ctrl Pts',(16.317900533139,6.,313.50573217442));
#10615=CARTESIAN_POINT('Ctrl Pts',(15.6278893738391,6.,313.517231811529));
#10616=CARTESIAN_POINT('Ctrl Pts',(14.2382065932492,6.,313.544340068234));
#10617=CARTESIAN_POINT('Ctrl Pts',(12.1247011523636,6.,313.597329370257));
#10618=CARTESIAN_POINT('Ctrl Pts',(9.24849377203438,6.,313.692736456781));
#10619=CARTESIAN_POINT('Ctrl Pts',(5.55693877490966,6.,313.853990642));
#10620=CARTESIAN_POINT('Ctrl Pts',(1.77365151465576,6.,314.058420030254));
#10621=CARTESIAN_POINT('Ctrl Pts',(-2.09023353797942,6.,314.307572958727));
#10622=CARTESIAN_POINT('Ctrl Pts',(-6.01421082656319,6.,314.603269922693));
#10623=CARTESIAN_POINT('Ctrl Pts',(-9.96528300844179,6.,314.947459907816));
#10624=CARTESIAN_POINT('Ctrl Pts',(-13.6094727938912,6.,315.313408028766));
#10625=CARTESIAN_POINT('Ctrl Pts',(-16.408608787372,6.,315.634868750851));
#10626=CARTESIAN_POINT('Ctrl Pts',(-18.3821515018489,6.,315.886718461855));
#10627=CARTESIAN_POINT('Ctrl Pts',(-19.579383939224,6.,316.050546317275));
#10628=CARTESIAN_POINT('Ctrl Pts',(-20.0405545273386,6.,316.115431789383));
#10629=CARTESIAN_POINT('',(16.317900533139,-6.,313.50573217442));
#10630=CARTESIAN_POINT('',(16.317900533139,-13.,313.50573217442));
#10631=CARTESIAN_POINT('',(-20.0405545265874,-6.,316.115431789172));
#10632=CARTESIAN_POINT('Ctrl Pts',(-20.0405545265728,-6.,316.115431789276));
#10633=CARTESIAN_POINT('Ctrl Pts',(-19.4004600929468,-6.,316.025372209181));
#10634=CARTESIAN_POINT('Ctrl Pts',(-18.7497721478954,-6.,315.937974131023));
#10635=CARTESIAN_POINT('Ctrl Pts',(-18.0906230620982,-6.00000000000001,
315.853146441753));
#10636=CARTESIAN_POINT('Ctrl Pts',(-17.5243686223842,-6.00000000000001,
315.780273617235));
#10637=CARTESIAN_POINT('Ctrl Pts',(-16.9518707527639,-6.00000000000001,
315.709298340212));
#10638=CARTESIAN_POINT('Ctrl Pts',(-16.3744431251552,-6.00000000000001,
315.640175937909));
#10639=CARTESIAN_POINT('Ctrl Pts',(-15.8474128379684,-6.00000000000001,
315.577086473887));
#10640=CARTESIAN_POINT('Ctrl Pts',(-15.3162762637607,-6.00000000000002,
315.515540826831));
#10641=CARTESIAN_POINT('Ctrl Pts',(-14.7819888683864,-6.00000000000002,
315.455511511763));
#10642=CARTESIAN_POINT('Ctrl Pts',(-14.2794448395025,-6.00000000000002,
315.399048690243));
#10643=CARTESIAN_POINT('Ctrl Pts',(-13.7741136098437,-6.00000000000002,
315.34392752094));
#10644=CARTESIAN_POINT('Ctrl Pts',(-13.2667442133851,-6.00000000000002,
315.290128438354));
#10645=CARTESIAN_POINT('Ctrl Pts',(-12.7800008415808,-6.00000000000002,
315.238516443147));
#10646=CARTESIAN_POINT('Ctrl Pts',(-12.2913818748689,-6.00000000000002,
315.188121314751));
#10647=CARTESIAN_POINT('Ctrl Pts',(-11.8015007656218,-6.00000000000003,
315.138927292701));
#10648=CARTESIAN_POINT('Ctrl Pts',(-11.3278770637046,-6.00000000000003,
315.09136584484));
#10649=CARTESIAN_POINT('Ctrl Pts',(-10.8530737841221,-6.00000000000003,
315.04492717112));
#10650=CARTESIAN_POINT('Ctrl Pts',(-10.3775966580326,-6.00000000000003,
314.999597383367));
#10651=CARTESIAN_POINT('Ctrl Pts',(-9.90819256207086,-6.00000000000003,
314.954846570189));
#10652=CARTESIAN_POINT('Ctrl Pts',(-9.43813190999691,-6.00000000000004,
314.91117654094));
#10653=CARTESIAN_POINT('Ctrl Pts',(-8.96784969603263,-6.00000000000004,
314.868573440465));
#10654=CARTESIAN_POINT('Ctrl Pts',(-8.48876740980112,-6.00000000000004,
314.825173137051));
#10655=CARTESIAN_POINT('Ctrl Pts',(-8.00945507896517,-6.00000000000004,
314.782880048696));
#10656=CARTESIAN_POINT('Ctrl Pts',(-7.53031845791347,-6.00000000000004,
314.74167888733));
#10657=CARTESIAN_POINT('Ctrl Pts',(-7.04087742046235,-6.00000000000004,
314.699591644826));
#10658=CARTESIAN_POINT('Ctrl Pts',(-6.55161960647171,-6.00000000000004,
314.658643780709));
#10659=CARTESIAN_POINT('Ctrl Pts',(-6.06292338188131,-6.00000000000005,
314.61881862178));
#10660=CARTESIAN_POINT('Ctrl Pts',(-5.55931863250807,-6.00000000000005,
314.577778527398));
#10661=CARTESIAN_POINT('Ctrl Pts',(-5.05631021845046,-6.00000000000005,
314.53793066474));
#10662=CARTESIAN_POINT('Ctrl Pts',(-4.5542566466415,-6.00000000000005,314.499256707419));
#10663=CARTESIAN_POINT('Ctrl Pts',(-4.04238010851235,-6.00000000000005,
314.459826071923));
#10664=CARTESIAN_POINT('Ctrl Pts',(-3.5314960243371,-6.00000000000005,314.42161571284));
#10665=CARTESIAN_POINT('Ctrl Pts',(-3.0219286923217,-6.00000000000006,314.384606361902));
#10666=CARTESIAN_POINT('Ctrl Pts',(-2.50115143391243,-6.00000000000006,
314.346782845546));
#10667=CARTESIAN_POINT('Ctrl Pts',(-1.98174936982304,-6.00000000000006,
314.310213743213));
#10668=CARTESIAN_POINT('Ctrl Pts',(-1.46401295479278,-6.00000000000006,
314.274878890499));
#10669=CARTESIAN_POINT('Ctrl Pts',(-0.933109127184629,-6.00000000000006,
314.238645378602));
#10670=CARTESIAN_POINT('Ctrl Pts',(-0.403956593770315,-6.00000000000006,
314.203709674355));
#10671=CARTESIAN_POINT('Ctrl Pts',(0.123187284072103,-6.00000000000006,
314.170050747481));
#10672=CARTESIAN_POINT('Ctrl Pts',(0.665680905887875,-6.00000000000007,
314.135411716443));
#10673=CARTESIAN_POINT('Ctrl Pts',(1.20604737288525,-6.00000000000007,314.102124875805));
#10674=CARTESIAN_POINT('Ctrl Pts',(1.74406199402793,-6.00000000000007,314.070168409682));
#10675=CARTESIAN_POINT('Ctrl Pts',(2.29915491822338,-6.00000000000007,314.037197543222));
#10676=CARTESIAN_POINT('Ctrl Pts',(2.85174452453734,-6.00000000000007,314.00564282438));
#10677=CARTESIAN_POINT('Ctrl Pts',(3.40163952961782,-6.00000000000008,313.975481885011));
#10678=CARTESIAN_POINT('Ctrl Pts',(3.98358848909718,-6.00000000000008,313.943562832973));
#10679=CARTESIAN_POINT('Ctrl Pts',(4.56251959828842,-6.00000000000008,313.913204744328));
#10680=CARTESIAN_POINT('Ctrl Pts',(5.13826572536412,-6.00000000000008,313.884383410908));
#10681=CARTESIAN_POINT('Ctrl Pts',(5.73956593775672,-6.00000000000008,313.854282862954));
#10682=CARTESIAN_POINT('Ctrl Pts',(6.33739249073037,-6.00000000000009,313.8258584665));
#10683=CARTESIAN_POINT('Ctrl Pts',(6.93161508868178,-6.00000000000009,313.799085785577));
#10684=CARTESIAN_POINT('Ctrl Pts',(7.55902819791957,-6.00000000000009,313.770817707187));
#10685=CARTESIAN_POINT('Ctrl Pts',(8.18242392403445,-6.00000000000009,313.744390948001));
#10686=CARTESIAN_POINT('Ctrl Pts',(8.80170884735432,-6.00000000000009,313.71978104624));
#10687=CARTESIAN_POINT('Ctrl Pts',(9.50347615746683,-6.0000000000001,313.691893358505));
#10688=CARTESIAN_POINT('Ctrl Pts',(10.1999648801093,-6.0000000000001,313.666338546755));
#10689=CARTESIAN_POINT('Ctrl Pts',(10.8911103594156,-6.0000000000001,313.643088515844));
#10690=CARTESIAN_POINT('Ctrl Pts',(11.670124147706,-6.0000000000001,313.616882608115));
#10691=CARTESIAN_POINT('Ctrl Pts',(12.44235109068,-6.00000000000011,313.593604477312));
#10692=CARTESIAN_POINT('Ctrl Pts',(13.2077719903083,-6.00000000000011,313.573226843001));
#10693=CARTESIAN_POINT('Ctrl Pts',(14.2572610604321,-6.00000000000011,313.545286523506));
#10694=CARTESIAN_POINT('Ctrl Pts',(15.2939614463516,-6.00000000000012,313.522797011359));
#10695=CARTESIAN_POINT('Ctrl Pts',(16.317900533139,-6.00000000000012,313.50573217442));
#10696=CARTESIAN_POINT('',(-34.7643786318829,-6.,326.55931644625));
#10697=CARTESIAN_POINT('Ctrl Pts',(-20.0405545265728,-6.,316.115431789276));
#10698=CARTESIAN_POINT('Ctrl Pts',(-20.7549729434527,-6.,316.21594855564));
#10699=CARTESIAN_POINT('Ctrl Pts',(-21.4561906038213,-6.,316.319779472749));
#10700=CARTESIAN_POINT('Ctrl Pts',(-22.1412177785273,-6.,316.427092714018));
#10701=CARTESIAN_POINT('Ctrl Pts',(-22.6934545573852,-6.,316.513603615885));
#10702=CARTESIAN_POINT('Ctrl Pts',(-23.2351674585656,-6.,316.602378254545));
#10703=CARTESIAN_POINT('Ctrl Pts',(-23.7648154461404,-6.,316.693530260689));
#10704=CARTESIAN_POINT('Ctrl Pts',(-24.2381920307505,-6.,316.77499800221));
#10705=CARTESIAN_POINT('Ctrl Pts',(-24.7019304370803,-6.,316.858364961178));
#10706=CARTESIAN_POINT('Ctrl Pts',(-25.1549683114691,-6.,316.943730630041));
#10707=CARTESIAN_POINT('Ctrl Pts',(-25.5795553714899,-6.,317.023735328143));
#10708=CARTESIAN_POINT('Ctrl Pts',(-25.9947432901691,-6.,317.10549566778));
#10709=CARTESIAN_POINT('Ctrl Pts',(-26.3997003202801,-6.,317.189109078339));
#10710=CARTESIAN_POINT('Ctrl Pts',(-26.7856515095121,-6.,317.268798262232));
#10711=CARTESIAN_POINT('Ctrl Pts',(-27.1623093224257,-6.,317.350170711296));
#10712=CARTESIAN_POINT('Ctrl Pts',(-27.5289986025995,-6.,317.433324389979));
#10713=CARTESIAN_POINT('Ctrl Pts',(-27.8785558810865,-6.,317.512593065636));
#10714=CARTESIAN_POINT('Ctrl Pts',(-28.2190541342782,-6.,317.593480454025));
#10715=CARTESIAN_POINT('Ctrl Pts',(-28.5499534894729,-6.,317.676083421344));
#10716=CARTESIAN_POINT('Ctrl Pts',(-28.8655920291323,-6.,317.754876805395));
#10717=CARTESIAN_POINT('Ctrl Pts',(-29.1724963802546,-6.,317.835231170493));
#10718=CARTESIAN_POINT('Ctrl Pts',(-29.4702436223019,-6.,317.917241665508));
#10719=CARTESIAN_POINT('Ctrl Pts',(-29.7569275835638,-6.,317.996204927819));
#10720=CARTESIAN_POINT('Ctrl Pts',(-30.035122074916,-6.,318.076703525759));
#10721=CARTESIAN_POINT('Ctrl Pts',(-30.304496360236,-6.,318.158833019446));
#10722=CARTESIAN_POINT('Ctrl Pts',(-30.5702374847235,-6.,318.239854799161));
#10723=CARTESIAN_POINT('Ctrl Pts',(-30.8273945384287,-6.,318.322463785503));
#10724=CARTESIAN_POINT('Ctrl Pts',(-31.0757000696003,-6.,318.406762502099));
#10725=CARTESIAN_POINT('Ctrl Pts',(-31.324823150672,-6.,318.491338773558));
#10726=CARTESIAN_POINT('Ctrl Pts',(-31.5650363297957,-6.,318.577616001022));
#10727=CARTESIAN_POINT('Ctrl Pts',(-31.7961210268803,-6.,318.665707788871));
#10728=CARTESIAN_POINT('Ctrl Pts',(-32.0279623515194,-6.,318.754088010679));
#10729=CARTESIAN_POINT('Ctrl Pts',(-32.2506153233891,-6.,318.844294777607));
#10730=CARTESIAN_POINT('Ctrl Pts',(-32.4639109145767,-6.,318.936451698723));
#10731=CARTESIAN_POINT('Ctrl Pts',(-32.6810137977926,-6.,319.030253606071));
#10732=CARTESIAN_POINT('Ctrl Pts',(-32.888422294495,-6.,319.126076024321));
#10733=CARTESIAN_POINT('Ctrl Pts',(-33.0860121094894,-6.,319.224057177318));
#10734=CARTESIAN_POINT('Ctrl Pts',(-33.297622908898,-6.,319.328991078457));
#10735=CARTESIAN_POINT('Ctrl Pts',(-33.4979721328517,-6.,319.436401195976));
#10736=CARTESIAN_POINT('Ctrl Pts',(-33.6869681337662,-6.,319.546463366874));
#10737=CARTESIAN_POINT('Ctrl Pts',(-33.8864368406078,-6.,319.662624337449));
#10738=CARTESIAN_POINT('Ctrl Pts',(-34.0732596226775,-6.,319.78173982131));
#10739=CARTESIAN_POINT('Ctrl Pts',(-34.2473912238251,-6.,319.90401788643));
#10740=CARTESIAN_POINT('Ctrl Pts',(-34.4306171129455,-6.,320.03268210966));
#10741=CARTESIAN_POINT('Ctrl Pts',(-34.5997920592249,-6.,320.164848461445));
#10742=CARTESIAN_POINT('Ctrl Pts',(-34.7549231941343,-6.,320.300752983988));
#10743=CARTESIAN_POINT('Ctrl Pts',(-34.9175912336802,-6.,320.443260303749));
#10744=CARTESIAN_POINT('Ctrl Pts',(-35.0648183398604,-6.,320.589878647392));
#10745=CARTESIAN_POINT('Ctrl Pts',(-35.1966684463826,-6.,320.740862499649));
#10746=CARTESIAN_POINT('Ctrl Pts',(-35.3331200653272,-6.,320.897115623886));
#10747=CARTESIAN_POINT('Ctrl Pts',(-35.4531036891042,-6.,321.058045238222));
#10748=CARTESIAN_POINT('Ctrl Pts',(-35.5567351883284,-6.,321.223901152682));
#10749=CARTESIAN_POINT('Ctrl Pts',(-35.666164567533,-6.,321.39903622158));
#10750=CARTESIAN_POINT('Ctrl Pts',(-35.7573622522126,-6.,321.579665476576));
#10751=CARTESIAN_POINT('Ctrl Pts',(-35.83049571681,-6.,321.766030282812));
#10752=CARTESIAN_POINT('Ctrl Pts',(-35.8990144606402,-6.,321.940635471939));
#10753=CARTESIAN_POINT('Ctrl Pts',(-35.9516781792488,-6.,322.120275264076));
#10754=CARTESIAN_POINT('Ctrl Pts',(-35.9886301568112,-6.,322.305095435263));
#10755=CARTESIAN_POINT('Ctrl Pts',(-36.0272612985265,-6.,322.498314166599));
#10756=CARTESIAN_POINT('Ctrl Pts',(-36.0487207806161,-6.,322.697194451537));
#10757=CARTESIAN_POINT('Ctrl Pts',(-36.0531635744342,-6.,322.901842878652));
#10758=CARTESIAN_POINT('Ctrl Pts',(-36.0578748107463,-6.,323.1188565733));
#10759=CARTESIAN_POINT('Ctrl Pts',(-36.0434514023682,-6.,323.342355832864));
#10760=CARTESIAN_POINT('Ctrl Pts',(-36.0100610340838,-6.,323.572410184283));
#10761=CARTESIAN_POINT('Ctrl Pts',(-35.9748650024435,-6.,323.814905270369));
#10762=CARTESIAN_POINT('Ctrl Pts',(-35.9185960651917,-6.,324.064682754654));
#10763=CARTESIAN_POINT('Ctrl Pts',(-35.8414212830246,-6.,324.321774846627));
#10764=CARTESIAN_POINT('Ctrl Pts',(-35.7641383003919,-6.,324.579227386447));
#10765=CARTESIAN_POINT('Ctrl Pts',(-35.6658915658653,-6.,324.844013841787));
#10766=CARTESIAN_POINT('Ctrl Pts',(-35.5468077850159,-6.,325.1161343829));
#10767=CARTESIAN_POINT('Ctrl Pts',(-35.4304704895933,-6.,325.381978879573));
#10768=CARTESIAN_POINT('Ctrl Pts',(-35.2942465138308,-6.,325.654821759961));
#10769=CARTESIAN_POINT('Ctrl Pts',(-35.1382069832313,-6.,325.934651028931));
#10770=CARTESIAN_POINT('Ctrl Pts',(-35.0241772447393,-6.,326.139143174226));
#10771=CARTESIAN_POINT('Ctrl Pts',(-34.8995644267643,-6.,326.347365946528));
#10772=CARTESIAN_POINT('Ctrl Pts',(-34.764378631884,-6.,326.559316446249));
#10773=CARTESIAN_POINT('',(-34.7643786318829,-13.,326.55931644625));
#10774=CARTESIAN_POINT('Origin',(-34.7643786318829,-13.,326.55931644625));
#10775=CARTESIAN_POINT('',(-33.0349479481876,6.,325.551079813359));
#10776=CARTESIAN_POINT('',(-33.0349479481876,-13.,325.551079813359));
#10777=CARTESIAN_POINT('',(-33.0349479481876,6.,325.551079813359));
#10778=CARTESIAN_POINT('Origin',(-9.91234501254369,-6.,320.032524310335));
#10779=CARTESIAN_POINT('',(-20.0407500733448,-6.,318.135777164329));
#10780=CARTESIAN_POINT('',(-20.0405545273386,-6.,325.214166745933));
#10781=CARTESIAN_POINT('',(-33.0349479481876,-6.,325.551079813359));
#10782=CARTESIAN_POINT('Ctrl Pts',(-33.0349479481876,-6.,325.551079813359));
#10783=CARTESIAN_POINT('Ctrl Pts',(-33.6174796157523,-6.,324.651156195591));
#10784=CARTESIAN_POINT('Ctrl Pts',(-33.9167172498653,-6.,323.906208160949));
#10785=CARTESIAN_POINT('Ctrl Pts',(-34.1037191682109,-6.,322.90805366785));
#10786=CARTESIAN_POINT('Ctrl Pts',(-34.0551194507184,-6.,322.664546739217));
#10787=CARTESIAN_POINT('Ctrl Pts',(-33.8035173417139,-6.,322.149720287837));
#10788=CARTESIAN_POINT('Ctrl Pts',(-33.5337647985207,-6.,321.817374523001));
#10789=CARTESIAN_POINT('Ctrl Pts',(-32.1374388202749,-6.,320.916078087379));
#10790=CARTESIAN_POINT('Ctrl Pts',(-30.8059455281908,-6.,320.365993587133));
#10791=CARTESIAN_POINT('Ctrl Pts',(-26.6717920677378,-6.,319.212778873305));
#10792=CARTESIAN_POINT('Ctrl Pts',(-23.5366870472917,-6.,318.635027950995));
#10793=CARTESIAN_POINT('Ctrl Pts',(-20.040945619351,-6.,318.135786350546));
#10794=CARTESIAN_POINT('',(-24.0704398622791,-6.,320.324882814963));
#10795=CARTESIAN_POINT('Ctrl Pts',(-33.0349479481876,-13.,325.551079813359));
#10796=CARTESIAN_POINT('Ctrl Pts',(-33.0349479481876,9.8,325.551079813359));
#10797=CARTESIAN_POINT('Ctrl Pts',(-33.6174796157523,-13.,324.651156195591));
#10798=CARTESIAN_POINT('Ctrl Pts',(-33.6174796157523,9.8,324.651156195591));
#10799=CARTESIAN_POINT('Ctrl Pts',(-33.9167172498653,-13.,323.906208160949));
#10800=CARTESIAN_POINT('Ctrl Pts',(-33.9167172498653,9.8,323.906208160949));
#10801=CARTESIAN_POINT('Ctrl Pts',(-34.0125475629435,-13.,323.394697592393));
#10802=CARTESIAN_POINT('Ctrl Pts',(-34.0125475629435,9.8,323.394697592393));
#10803=CARTESIAN_POINT('Ctrl Pts',(-34.1037191682109,-13.,322.90805366785));
#10804=CARTESIAN_POINT('Ctrl Pts',(-34.1037191682109,9.8,322.90805366785));
#10805=CARTESIAN_POINT('Ctrl Pts',(-34.0551194507184,-13.,322.664546739217));
#10806=CARTESIAN_POINT('Ctrl Pts',(-34.0551194507184,9.8,322.664546739217));
#10807=CARTESIAN_POINT('Ctrl Pts',(-33.9292861005445,-13.,322.407067430352));
#10808=CARTESIAN_POINT('Ctrl Pts',(-33.9292861005445,9.8,322.407067430352));
#10809=CARTESIAN_POINT('Ctrl Pts',(-33.8035173417139,-13.,322.149720287837));
#10810=CARTESIAN_POINT('Ctrl Pts',(-33.8035173417139,9.8,322.149720287837));
#10811=CARTESIAN_POINT('Ctrl Pts',(-33.5337647985207,-13.,321.817374523001));
#10812=CARTESIAN_POINT('Ctrl Pts',(-33.5337647985207,9.8,321.817374523001));
#10813=CARTESIAN_POINT('Ctrl Pts',(-32.9271647914283,-13.,321.425828112808));
#10814=CARTESIAN_POINT('Ctrl Pts',(-32.9271647914283,9.8,321.425828112808));
#10815=CARTESIAN_POINT('Ctrl Pts',(-32.1374388202749,-13.,320.916078087379));
#10816=CARTESIAN_POINT('Ctrl Pts',(-32.1374388202749,9.8,320.916078087379));
#10817=CARTESIAN_POINT('Ctrl Pts',(-30.8059455281908,-13.,320.365993587133));
#10818=CARTESIAN_POINT('Ctrl Pts',(-30.8059455281908,9.8,320.365993587133));
#10819=CARTESIAN_POINT('Ctrl Pts',(-29.043009016516,-13.,319.874225600227));
#10820=CARTESIAN_POINT('Ctrl Pts',(-29.043009016516,9.8,319.874225600227));
#10821=CARTESIAN_POINT('Ctrl Pts',(-25.8730053780895,-13.,318.989958754863));
#10822=CARTESIAN_POINT('Ctrl Pts',(-25.8730053780895,9.8,318.989958754863));
#10823=CARTESIAN_POINT('Ctrl Pts',(-21.3377690810308,-13.,318.255274354999));
#10824=CARTESIAN_POINT('Ctrl Pts',(-21.3377690810308,9.8,318.255274354999));
#10825=CARTESIAN_POINT('Ctrl Pts',(-16.4007776292659,-13.,317.65778048784));
#10826=CARTESIAN_POINT('Ctrl Pts',(-16.4007776292659,9.8,317.65778048784));
#10827=CARTESIAN_POINT('Ctrl Pts',(-11.7424615555448,-13.,317.094012996539));
#10828=CARTESIAN_POINT('Ctrl Pts',(-11.7424615555448,9.8,317.094012996539));
#10829=CARTESIAN_POINT('Ctrl Pts',(-6.76571504745064,-13.,316.650544330241));
#10830=CARTESIAN_POINT('Ctrl Pts',(-6.76571504745064,9.8,316.650544330241));
#10831=CARTESIAN_POINT('Ctrl Pts',(-1.96541115088432,-13.,316.314322154425));
#10832=CARTESIAN_POINT('Ctrl Pts',(-1.96541115088432,9.8,316.314322154425));
#10833=CARTESIAN_POINT('Ctrl Pts',(4.47207810420708,-13.,315.86342848378));
#10834=CARTESIAN_POINT('Ctrl Pts',(4.47207810420708,9.8,315.86342848378));
#10835=CARTESIAN_POINT('Ctrl Pts',(10.6153256845702,-13.,315.601684449612));
#10836=CARTESIAN_POINT('Ctrl Pts',(10.6153256845702,9.8,315.601684449612));
#10837=CARTESIAN_POINT('Ctrl Pts',(16.3179005331389,-13.,315.506011760182));
#10838=CARTESIAN_POINT('Ctrl Pts',(16.3179005331389,9.8,315.506011760182));
#10839=CARTESIAN_POINT('',(-33.0349479481876,-13.,325.551079813359));
#10840=CARTESIAN_POINT('',(16.3179005331391,-6.,315.506011760182));
#10841=CARTESIAN_POINT('Ctrl Pts',(16.3179005331389,-6.00000000000013,315.506011760182));
#10842=CARTESIAN_POINT('Ctrl Pts',(10.6153256845702,-6.00000000000013,315.601684449612));
#10843=CARTESIAN_POINT('Ctrl Pts',(4.47207810420708,-6.00000000000014,315.86342848378));
#10844=CARTESIAN_POINT('Ctrl Pts',(-6.76571504745064,-6.00000000000014,
316.650544330241));
#10845=CARTESIAN_POINT('Ctrl Pts',(-11.7424615555448,-6.00000000000014,
317.094012996539));
#10846=CARTESIAN_POINT('Ctrl Pts',(-17.6447244400945,-6.00000000000013,
317.808327758947));
#10847=CARTESIAN_POINT('Ctrl Pts',(-18.8631653699184,-6.00000000000013,
317.967584726398));
#10848=CARTESIAN_POINT('Ctrl Pts',(-20.0406883873031,-6.00000000000013,
318.135749614386));
#10849=CARTESIAN_POINT('',(16.3179005331391,6.,315.506011760182));
#10850=CARTESIAN_POINT('',(16.3179005331391,-13.,315.506011760182));
#10851=CARTESIAN_POINT('',(-20.0407500724488,6.00000000000001,318.135777164115));
#10852=CARTESIAN_POINT('Ctrl Pts',(-20.0406883866898,6.00000000000001,318.135749614298));
#10853=CARTESIAN_POINT('Ctrl Pts',(-18.8631653694953,6.00000000000001,317.967584726343));
#10854=CARTESIAN_POINT('Ctrl Pts',(-17.6447244398786,6.00000000000001,317.808327758921));
#10855=CARTESIAN_POINT('Ctrl Pts',(-11.7424615555448,6.00000000000001,317.094012996539));
#10856=CARTESIAN_POINT('Ctrl Pts',(-6.76571504745064,6.00000000000001,316.650544330241));
#10857=CARTESIAN_POINT('Ctrl Pts',(4.4720781042072,6.,315.86342848378));
#10858=CARTESIAN_POINT('Ctrl Pts',(10.6153256845705,6.,315.601684449612));
#10859=CARTESIAN_POINT('Ctrl Pts',(16.3179005331392,6.,315.506011760182));
#10860=CARTESIAN_POINT('Ctrl Pts',(-33.0349479481876,6.,325.551079813359));
#10861=CARTESIAN_POINT('Ctrl Pts',(-33.6174796157523,6.,324.651156195591));
#10862=CARTESIAN_POINT('Ctrl Pts',(-33.9167172498653,6.,323.906208160949));
#10863=CARTESIAN_POINT('Ctrl Pts',(-34.1037191682109,6.,322.90805366785));
#10864=CARTESIAN_POINT('Ctrl Pts',(-34.0551194507184,6.00000000000001,322.664546739217));
#10865=CARTESIAN_POINT('Ctrl Pts',(-33.8035173417139,6.00000000000001,322.149720287837));
#10866=CARTESIAN_POINT('Ctrl Pts',(-33.5337647985207,6.00000000000001,321.817374523001));
#10867=CARTESIAN_POINT('Ctrl Pts',(-32.1374388202749,6.00000000000001,320.916078087379));
#10868=CARTESIAN_POINT('Ctrl Pts',(-30.8059455281908,6.00000000000001,320.365993587133));
#10869=CARTESIAN_POINT('Ctrl Pts',(-26.6717920673326,6.00000000000001,319.212778873192));
#10870=CARTESIAN_POINT('Ctrl Pts',(-23.5366870462203,6.00000000000001,318.635027950798));
#10871=CARTESIAN_POINT('Ctrl Pts',(-20.0409456175589,6.00000000000001,318.13578635029));
#10872=CARTESIAN_POINT('Origin',(-34.7643786318829,-13.,326.55931644625));
#10873=CARTESIAN_POINT('Origin',(-9.91234501254369,6.,320.032524310335));
#10874=CARTESIAN_POINT('',(-20.0405545273386,6.,325.214166745933));
#10875=CARTESIAN_POINT('Origin',(-2.11984264684888,6.,322.999388292511));
#10876=CARTESIAN_POINT('',(16.317900533139,6.,326.637882383191));
#10877=CARTESIAN_POINT('',(16.317900533139,6.,315.999694146255));
#10878=CARTESIAN_POINT('',(-2.1198426468477,6.,336.998776585022));
#10879=CARTESIAN_POINT('Origin',(-2.35185291019846,6.,315.));
#10880=CARTESIAN_POINT('',(-20.0405545273386,6.,327.428945199355));
#10881=CARTESIAN_POINT('Origin',(-1.88783238349926,6.,315.));
#10882=CARTESIAN_POINT('',(-20.0405545273386,6.,325.214166745933));
#10883=CARTESIAN_POINT('',(-5.88783238349923,6.,328.556349186104));
#10884=CARTESIAN_POINT('Origin',(-1.88783238349926,6.,328.556349186104));
#10885=CARTESIAN_POINT('Origin',(-2.11984264684888,6.,322.999388292511));
#10886=CARTESIAN_POINT('',(-20.0405545273386,6.,325.214166745933));
#10887=CARTESIAN_POINT('',(16.317900533139,6.,315.999694146255));
#10888=CARTESIAN_POINT('Origin',(-20.0405545273386,-22.,327.428945199355));
#10889=CARTESIAN_POINT('',(-20.0405545273386,8.,327.428945199355));
#10890=CARTESIAN_POINT('',(-20.0405545273386,6.,327.428945199355));
#10891=CARTESIAN_POINT('',(-20.0405545273386,8.,325.214166745933));
#10892=CARTESIAN_POINT('Origin',(-2.11984264684888,8.,322.999388292511));
#10893=CARTESIAN_POINT('',(16.317900533139,8.,326.637882383191));
#10894=CARTESIAN_POINT('',(16.317900533139,8.,315.999694146255));
#10895=CARTESIAN_POINT('',(-2.1198426468477,8.,336.998776585022));
#10896=CARTESIAN_POINT('Origin',(-1.88783238349926,8.,315.));
#10897=CARTESIAN_POINT('Origin',(-2.35185291019846,8.,315.));
#10898=CARTESIAN_POINT('',(-5.88783238349923,8.,328.556349186104));
#10899=CARTESIAN_POINT('Origin',(-1.88783238349926,8.,328.556349186104));
#10900=CARTESIAN_POINT('Origin',(-1.88783238349926,6.,328.556349186104));
#10901=CARTESIAN_POINT('',(-5.88783238349923,6.,328.556349186104));
#10902=CARTESIAN_POINT('Origin',(-1.88783238349926,6.,315.));
#10903=CARTESIAN_POINT('',(-2.1198426468477,6.,336.998776585022));
#10904=CARTESIAN_POINT('Origin',(-2.35185291019846,6.,315.));
#10905=CARTESIAN_POINT('',(16.317900533139,6.,326.637882383191));
#10906=CARTESIAN_POINT('Origin',(-2.11984264684888,-6.,322.999388292511));
#10907=CARTESIAN_POINT('',(16.317900533139,-6.,315.999694146255));
#10908=CARTESIAN_POINT('',(-20.0405545273386,-6.,325.214166745933));
#10909=CARTESIAN_POINT('Origin',(-2.11984264684888,-6.,322.999388292511));
#10910=CARTESIAN_POINT('',(-20.0405545273386,-6.,327.428945199355));
#10911=CARTESIAN_POINT('',(-20.0405545273386,-6.,325.214166745933));
#10912=CARTESIAN_POINT('',(-2.1198426468477,-6.,336.998776585022));
#10913=CARTESIAN_POINT('Origin',(-1.88783238349926,-6.,315.));
#10914=CARTESIAN_POINT('',(16.317900533139,-6.,326.637882383191));
#10915=CARTESIAN_POINT('Origin',(-2.35185291019846,-6.,315.));
#10916=CARTESIAN_POINT('',(16.317900533139,-6.,315.999694146255));
#10917=CARTESIAN_POINT('',(-5.88783238349923,-6.,328.556349186104));
#10918=CARTESIAN_POINT('Origin',(-1.88783238349926,-6.,328.556349186104));
#10919=CARTESIAN_POINT('Origin',(16.317900533139,-8.,309.));
#10920=CARTESIAN_POINT('',(16.317900533139,-8.,326.637882383191));
#10921=CARTESIAN_POINT('',(16.317900533139,-8.,326.637882383191));
#10922=CARTESIAN_POINT('',(16.317900533139,-8.,315.999694146255));
#10923=CARTESIAN_POINT('Origin',(-20.0405545273386,-8.,327.428945199355));
#10924=CARTESIAN_POINT('',(-20.0405545273386,-8.,327.428945199355));
#10925=CARTESIAN_POINT('',(-20.0405545273386,-8.,325.214166745933));
#10926=CARTESIAN_POINT('',(-20.0405545273386,-8.,327.428945199355));
#10927=CARTESIAN_POINT('Origin',(-1.88783238349926,-8.,328.556349186104));
#10928=CARTESIAN_POINT('',(-5.88783238349923,-8.,328.556349186104));
#10929=CARTESIAN_POINT('Origin',(-1.88783238349926,-8.,328.556349186104));
#10930=CARTESIAN_POINT('',(-5.88783238349923,-8.,328.556349186104));
#10931=CARTESIAN_POINT('Origin',(-1.88783238349926,-8.,315.));
#10932=CARTESIAN_POINT('',(-2.1198426468477,-8.,336.998776585022));
#10933=CARTESIAN_POINT('Origin',(-1.88783238349926,-8.,315.));
#10934=CARTESIAN_POINT('',(-2.1198426468477,-8.,336.998776585022));
#10935=CARTESIAN_POINT('Origin',(-2.35185291019846,-8.,315.));
#10936=CARTESIAN_POINT('Origin',(-2.35185291019846,-8.,315.));
#10937=CARTESIAN_POINT('Origin',(-2.11984264684888,-8.,322.999388292511));
#19428=UNCERTAINTY_MEASURE_WITH_UNIT(LENGTH_MEASURE(0.01),#19444,
'DISTANCE_ACCURACY_VALUE',
'Maximum model space distance between geometric entities at asserted c
onnectivities');
#19433=UNCERTAINTY_MEASURE_WITH_UNIT(LENGTH_MEASURE(0.01),#19444,
'DISTANCE_ACCURACY_VALUE',
'Maximum model space distance between geometric entities at asserted c
onnectivities');
#19438=(
GEOMETRIC_REPRESENTATION_CONTEXT(3)
GLOBAL_UNCERTAINTY_ASSIGNED_CONTEXT((#19428))
GLOBAL_UNIT_ASSIGNED_CONTEXT((#19444,#19446,#19447))
REPRESENTATION_CONTEXT('','3D')
);
#19443=(
GEOMETRIC_REPRESENTATION_CONTEXT(3)
GLOBAL_UNCERTAINTY_ASSIGNED_CONTEXT((#19433))
GLOBAL_UNIT_ASSIGNED_CONTEXT((#19444,#19446,#19447))
REPRESENTATION_CONTEXT('','3D')
);
#19444=(
LENGTH_UNIT()
NAMED_UNIT(*)
SI_UNIT(.MILLI.,.METRE.)
);
#19446=(
NAMED_UNIT(*)
PLANE_ANGLE_UNIT()
SI_UNIT($,.RADIAN.)
);
#19447=(
NAMED_UNIT(*)
SI_UNIT($,.STERADIAN.)
SOLID_ANGLE_UNIT()
);
#19452=SHAPE_DEFINITION_REPRESENTATION(#19461,#19478);
#19461=PRODUCT_DEFINITION_SHAPE('',$,#19488);
#19478=SHAPE_REPRESENTATION('',(#2150),#19438);
#19483=PRODUCT_DEFINITION_CONTEXT('part definition',#19512,'design');
#19488=PRODUCT_DEFINITION('Clamp','Clamp',#19497,#19483);
#19497=PRODUCT_DEFINITION_FORMATION('',$,#19518);
#19512=APPLICATION_CONTEXT(
'Core Data for Automotive Mechanical Design Process');
#19513=PRODUCT_CONTEXT('part definition',#19512,'mechanical');
#19518=PRODUCT('Clamp','Clamp',$,(#19513));
#19525=PRESENTATION_STYLE_ASSIGNMENT((#19528));
#19528=SURFACE_STYLE_USAGE(.BOTH.,#19531);
#19531=SURFACE_SIDE_STYLE('',(#19534));
#19534=SURFACE_STYLE_FILL_AREA(#19537);
#19537=FILL_AREA_STYLE('Opaque(160,160,160)',(#19540));
#19540=FILL_AREA_STYLE_COLOUR('Opaque(160,160,160)',#19543);
#19543=COLOUR_RGB('Opaque(160,160,160)',0.627450980392157,0.627450980392157,
0.627450980392157);
ENDSEC;
END-ISO-10303-21;
